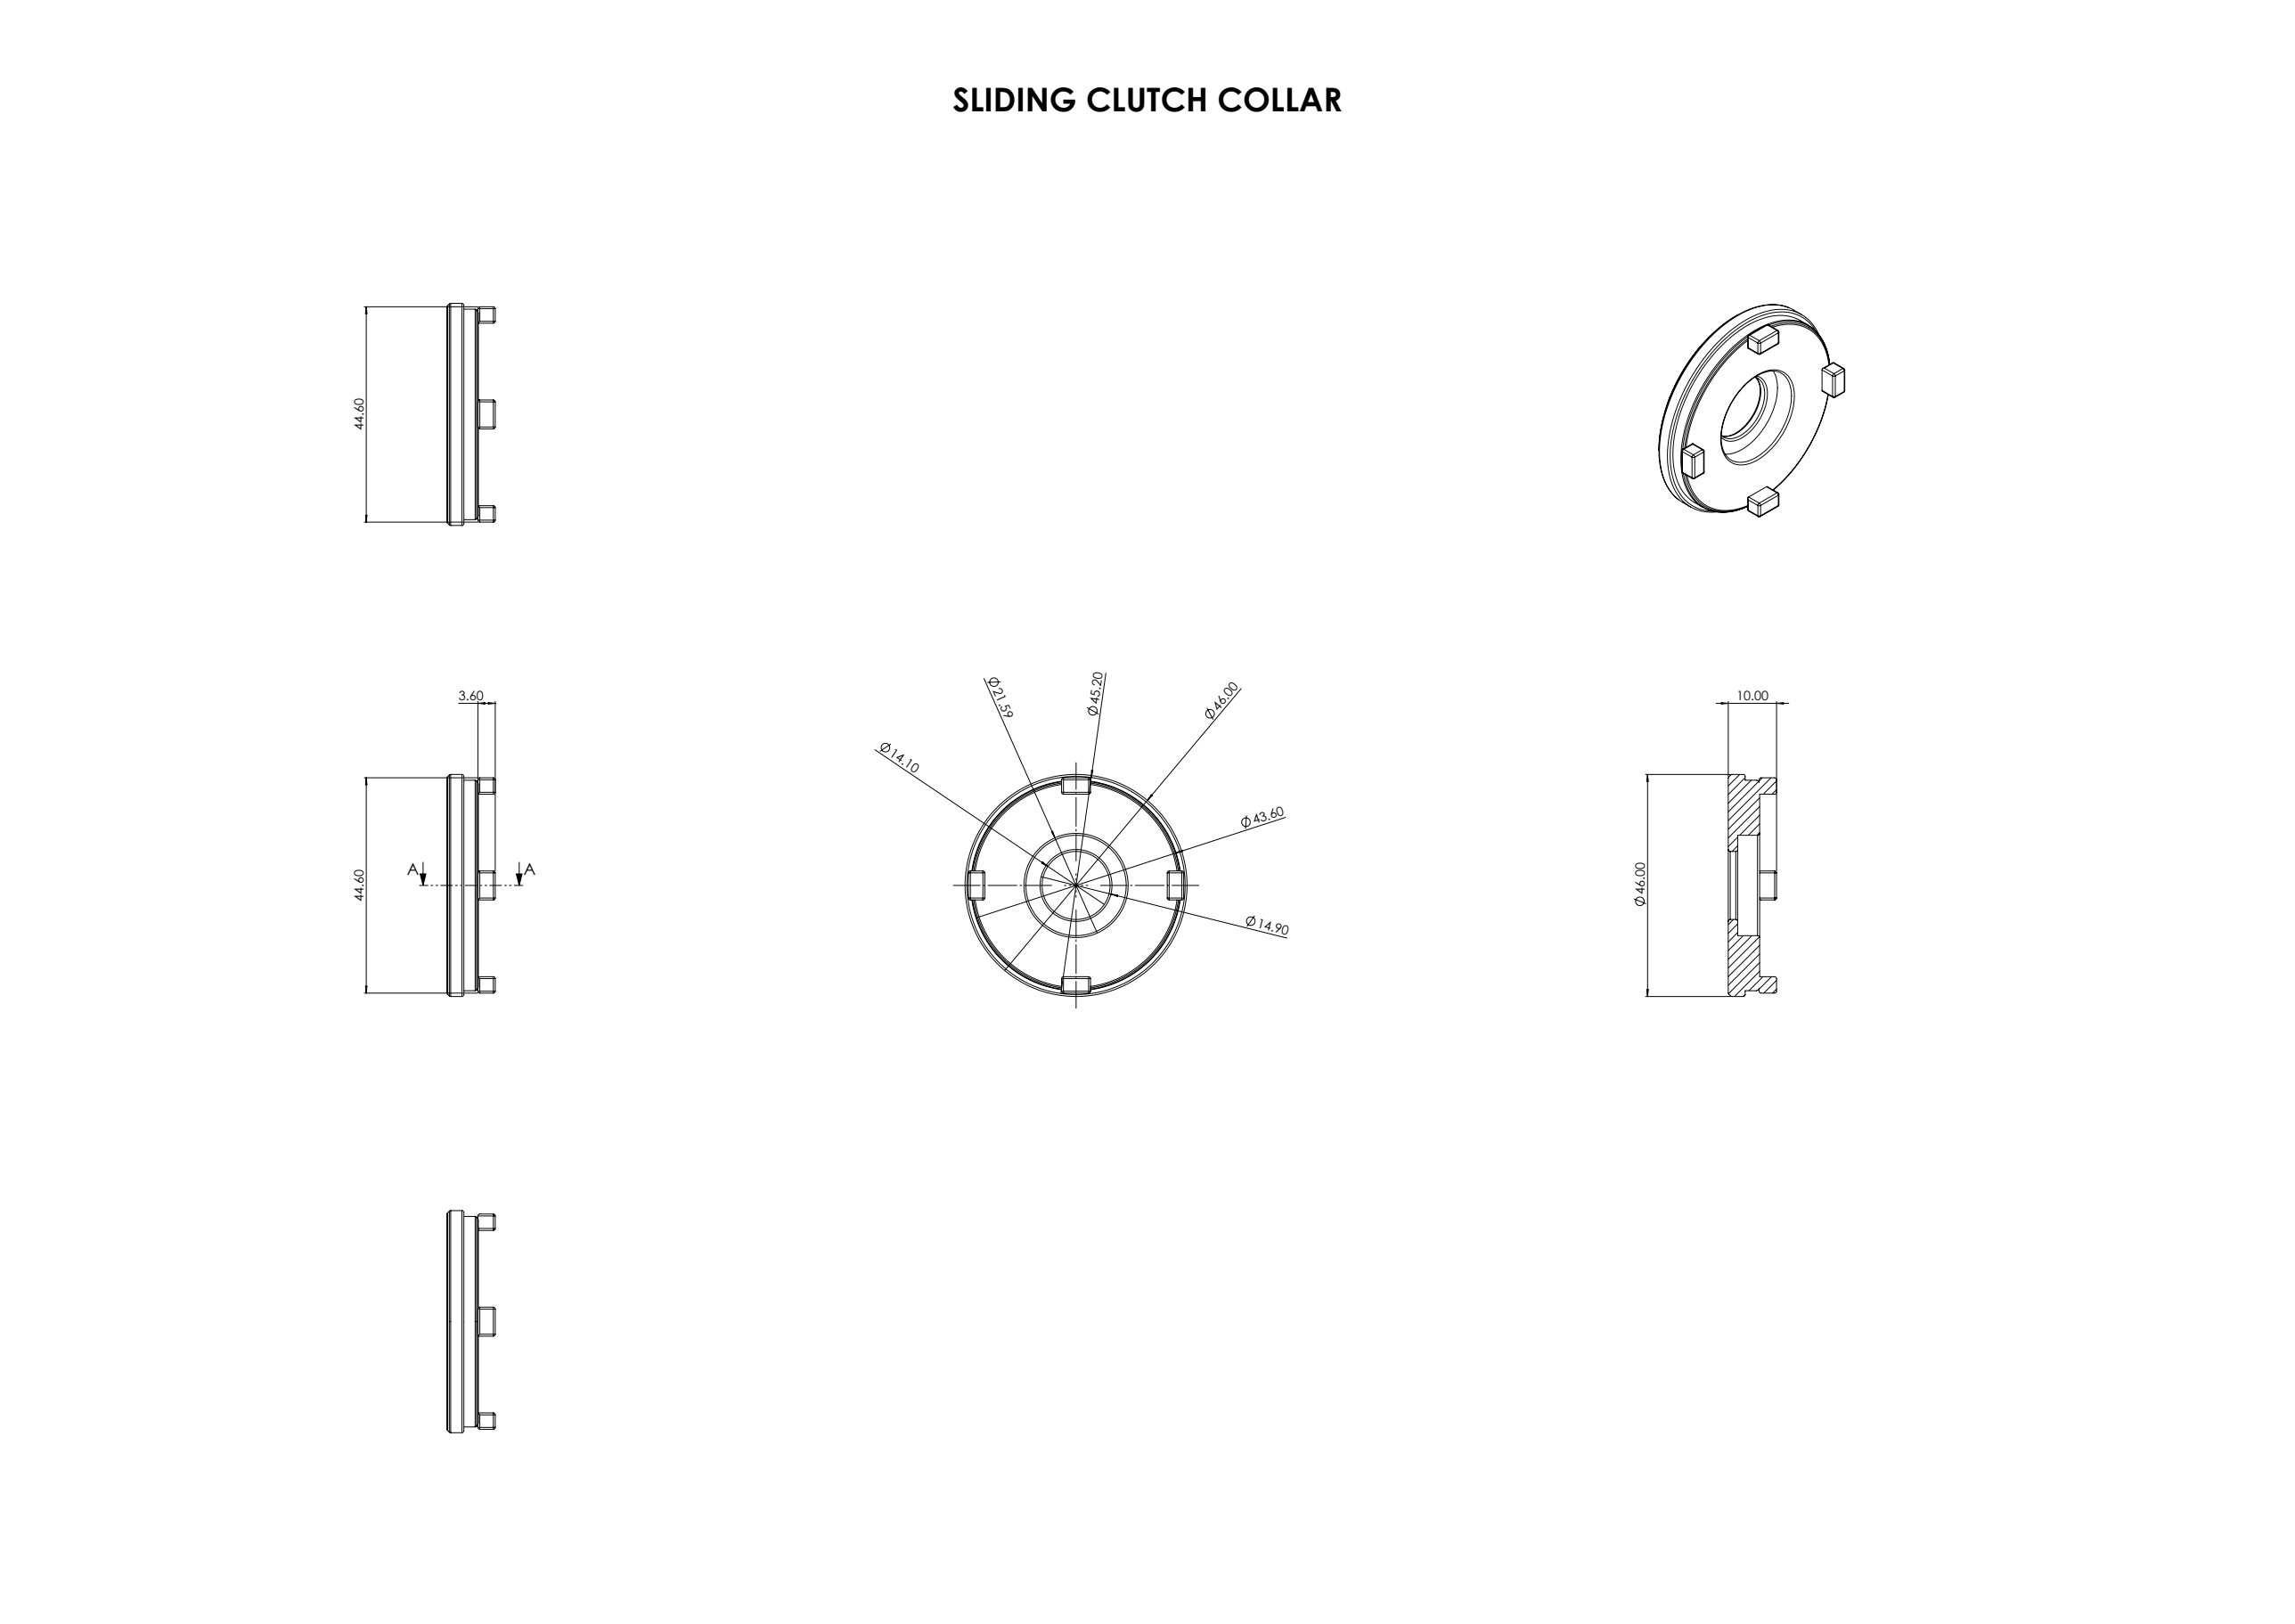
ISO-10303-21;
HEADER;
/* Generated by software containing ST-Developer
 * from STEP Tools, Inc. (www.steptools.com) 
 */

FILE_DESCRIPTION(
/* description */ (''),
/* implementation_level */ '2;1');

FILE_NAME(
/* name */ '08_Sliding_Clutch_Collar.step',
/* time_stamp */ '2026-10-11T13:00:10-07:00',
/* author */ (''),
/* organization */ (''),
/* preprocessor_version */ 'ST-DEVELOPER v20.2',
/* originating_system */ 'Autodesk Translation Framework v15.15.0.0',
/* authorisation */ '');

FILE_SCHEMA (('AUTOMOTIVE_DESIGN { 1 0 10303 214 3 1 1 }'));
ENDSEC;

DATA;
#10=MECHANICAL_DESIGN_GEOMETRIC_PRESENTATION_REPRESENTATION('',(#365),#65563);
#160=TOROIDAL_SURFACE('',#21892,21.1343145750508,0.4);
#161=TOROIDAL_SURFACE('',#21909,22.6,0.4);
#162=TOROIDAL_SURFACE('',#21951,22.6,0.4);
#163=TOROIDAL_SURFACE('',#21958,21.4,0.4);
#164=TOROIDAL_SURFACE('',#21963,10.7968626966597,0.4);
#165=TOROIDAL_SURFACE('',#21966,22.2343145750508,0.4);
#166=TOROIDAL_SURFACE('',#21990,7.45,0.4);
#167=TOROIDAL_SURFACE('',#21997,7.45,0.4);
#233=ELLIPSE('',#21780,0.565685424949238,0.4);
#234=ELLIPSE('',#21783,0.565685424949238,0.4);
#235=ELLIPSE('',#21819,0.565685424949238,0.4);
#236=ELLIPSE('',#21828,0.565685424949238,0.4);
#237=ELLIPSE('',#21872,0.565685424949238,0.4);
#238=ELLIPSE('',#21877,0.565685424949238,0.4);
#239=ELLIPSE('',#21929,0.565685424949238,0.4);
#240=ELLIPSE('',#21973,0.565685424949238,0.4);
#292=SPHERICAL_SURFACE('',#21784,0.4);
#293=SPHERICAL_SURFACE('',#21791,0.4);
#294=SPHERICAL_SURFACE('',#21794,0.4);
#295=SPHERICAL_SURFACE('',#21799,0.4);
#296=SPHERICAL_SURFACE('',#21809,0.4);
#297=SPHERICAL_SURFACE('',#21823,0.4);
#298=SPHERICAL_SURFACE('',#21831,0.4);
#299=SPHERICAL_SURFACE('',#21833,0.4);
#300=SPHERICAL_SURFACE('',#21840,0.4);
#301=SPHERICAL_SURFACE('',#21846,0.4);
#302=SPHERICAL_SURFACE('',#21859,0.4);
#303=SPHERICAL_SURFACE('',#21862,0.4);
#304=SPHERICAL_SURFACE('',#21879,0.4);
#305=SPHERICAL_SURFACE('',#21881,0.4);
#306=SPHERICAL_SURFACE('',#21919,0.4);
#307=SPHERICAL_SURFACE('',#21925,0.4);
#308=SPHERICAL_SURFACE('',#21937,0.4);
#309=SPHERICAL_SURFACE('',#21940,0.4);
#310=SPHERICAL_SURFACE('',#21942,0.4);
#311=SPHERICAL_SURFACE('',#21974,0.4);
#312=SPHERICAL_SURFACE('',#21982,0.4);
#313=SPHERICAL_SURFACE('',#21985,0.4);
#343=SHAPE_REPRESENTATION_RELATIONSHIP('SRR','None',#65621,#354);
#354=ADVANCED_BREP_SHAPE_REPRESENTATION('',(#376),#65559);
#365=STYLED_ITEM('',(#65802),#376);
#376=MANIFOLD_SOLID_BREP('Body1',#20015);
#493=CONICAL_SURFACE('',#21906,21.55,0.785398163397451);
#494=CONICAL_SURFACE('',#21955,22.7,0.785398163397452);
#984=PLANE('',#21804);
#985=PLANE('',#21805);
#986=PLANE('',#21814);
#987=PLANE('',#21815);
#988=PLANE('',#21838);
#989=PLANE('',#21852);
#990=PLANE('',#21853);
#991=PLANE('',#21869);
#992=PLANE('',#21885);
#993=PLANE('',#21886);
#994=PLANE('',#21888);
#995=PLANE('',#21902);
#996=PLANE('',#21917);
#997=PLANE('',#21926);
#998=PLANE('',#21927);
#999=PLANE('',#21944);
#1000=PLANE('',#21947);
#1001=PLANE('',#21950);
#1002=PLANE('',#21969);
#1003=PLANE('',#21978);
#1004=PLANE('',#21981);
#1005=PLANE('',#22000);
#1006=PLANE('',#22003);
#1007=PLANE('',#22004);
#1008=PLANE('',#22005);
#1009=PLANE('',#22006);
#1010=PLANE('',#22007);
#1011=PLANE('',#22008);
#1120=FACE_BOUND('',#3296,.T.);
#1121=FACE_BOUND('',#3301,.T.);
#1122=FACE_BOUND('',#3326,.T.);
#1123=FACE_BOUND('',#3342,.T.);
#2016=FACE_OUTER_BOUND('',#3240,.T.);
#2017=FACE_OUTER_BOUND('',#3241,.T.);
#2018=FACE_OUTER_BOUND('',#3242,.T.);
#2019=FACE_OUTER_BOUND('',#3243,.T.);
#2020=FACE_OUTER_BOUND('',#3244,.T.);
#2021=FACE_OUTER_BOUND('',#3245,.T.);
#2022=FACE_OUTER_BOUND('',#3246,.T.);
#2023=FACE_OUTER_BOUND('',#3247,.T.);
#2024=FACE_OUTER_BOUND('',#3248,.T.);
#2025=FACE_OUTER_BOUND('',#3249,.T.);
#2026=FACE_OUTER_BOUND('',#3250,.T.);
#2027=FACE_OUTER_BOUND('',#3251,.T.);
#2028=FACE_OUTER_BOUND('',#3252,.T.);
#2029=FACE_OUTER_BOUND('',#3253,.T.);
#2030=FACE_OUTER_BOUND('',#3254,.T.);
#2031=FACE_OUTER_BOUND('',#3255,.T.);
#2032=FACE_OUTER_BOUND('',#3256,.T.);
#2033=FACE_OUTER_BOUND('',#3257,.T.);
#2034=FACE_OUTER_BOUND('',#3258,.T.);
#2035=FACE_OUTER_BOUND('',#3259,.T.);
#2036=FACE_OUTER_BOUND('',#3260,.T.);
#2037=FACE_OUTER_BOUND('',#3261,.T.);
#2038=FACE_OUTER_BOUND('',#3262,.T.);
#2039=FACE_OUTER_BOUND('',#3263,.T.);
#2040=FACE_OUTER_BOUND('',#3264,.T.);
#2041=FACE_OUTER_BOUND('',#3265,.T.);
#2042=FACE_OUTER_BOUND('',#3266,.T.);
#2043=FACE_OUTER_BOUND('',#3267,.T.);
#2044=FACE_OUTER_BOUND('',#3268,.T.);
#2045=FACE_OUTER_BOUND('',#3269,.T.);
#2046=FACE_OUTER_BOUND('',#3270,.T.);
#2047=FACE_OUTER_BOUND('',#3271,.T.);
#2048=FACE_OUTER_BOUND('',#3272,.T.);
#2049=FACE_OUTER_BOUND('',#3273,.T.);
#2050=FACE_OUTER_BOUND('',#3274,.T.);
#2051=FACE_OUTER_BOUND('',#3275,.T.);
#2052=FACE_OUTER_BOUND('',#3276,.T.);
#2053=FACE_OUTER_BOUND('',#3277,.T.);
#2054=FACE_OUTER_BOUND('',#3278,.T.);
#2055=FACE_OUTER_BOUND('',#3279,.T.);
#2056=FACE_OUTER_BOUND('',#3280,.T.);
#2057=FACE_OUTER_BOUND('',#3281,.T.);
#2058=FACE_OUTER_BOUND('',#3282,.T.);
#2059=FACE_OUTER_BOUND('',#3283,.T.);
#2060=FACE_OUTER_BOUND('',#3284,.T.);
#2061=FACE_OUTER_BOUND('',#3285,.T.);
#2062=FACE_OUTER_BOUND('',#3286,.T.);
#2063=FACE_OUTER_BOUND('',#3287,.T.);
#2064=FACE_OUTER_BOUND('',#3288,.T.);
#2065=FACE_OUTER_BOUND('',#3289,.T.);
#2066=FACE_OUTER_BOUND('',#3290,.T.);
#2067=FACE_OUTER_BOUND('',#3291,.T.);
#2068=FACE_OUTER_BOUND('',#3292,.T.);
#2069=FACE_OUTER_BOUND('',#3293,.T.);
#2070=FACE_OUTER_BOUND('',#3294,.T.);
#2071=FACE_OUTER_BOUND('',#3295,.T.);
#2072=FACE_OUTER_BOUND('',#3297,.T.);
#2073=FACE_OUTER_BOUND('',#3298,.T.);
#2074=FACE_OUTER_BOUND('',#3299,.T.);
#2075=FACE_OUTER_BOUND('',#3300,.T.);
#2076=FACE_OUTER_BOUND('',#3302,.T.);
#2077=FACE_OUTER_BOUND('',#3303,.T.);
#2078=FACE_OUTER_BOUND('',#3304,.T.);
#2079=FACE_OUTER_BOUND('',#3305,.T.);
#2080=FACE_OUTER_BOUND('',#3306,.T.);
#2081=FACE_OUTER_BOUND('',#3307,.T.);
#2082=FACE_OUTER_BOUND('',#3308,.T.);
#2083=FACE_OUTER_BOUND('',#3309,.T.);
#2084=FACE_OUTER_BOUND('',#3310,.T.);
#2085=FACE_OUTER_BOUND('',#3311,.T.);
#2086=FACE_OUTER_BOUND('',#3312,.T.);
#2087=FACE_OUTER_BOUND('',#3313,.T.);
#2088=FACE_OUTER_BOUND('',#3314,.T.);
#2089=FACE_OUTER_BOUND('',#3315,.T.);
#2090=FACE_OUTER_BOUND('',#3316,.T.);
#2091=FACE_OUTER_BOUND('',#3317,.T.);
#2092=FACE_OUTER_BOUND('',#3318,.T.);
#2093=FACE_OUTER_BOUND('',#3319,.T.);
#2094=FACE_OUTER_BOUND('',#3320,.T.);
#2095=FACE_OUTER_BOUND('',#3321,.T.);
#2096=FACE_OUTER_BOUND('',#3322,.T.);
#2097=FACE_OUTER_BOUND('',#3323,.T.);
#2098=FACE_OUTER_BOUND('',#3324,.T.);
#2099=FACE_OUTER_BOUND('',#3325,.T.);
#2100=FACE_OUTER_BOUND('',#3327,.T.);
#2101=FACE_OUTER_BOUND('',#3328,.T.);
#2102=FACE_OUTER_BOUND('',#3329,.T.);
#2103=FACE_OUTER_BOUND('',#3330,.T.);
#2104=FACE_OUTER_BOUND('',#3331,.T.);
#2105=FACE_OUTER_BOUND('',#3332,.T.);
#2106=FACE_OUTER_BOUND('',#3333,.T.);
#2107=FACE_OUTER_BOUND('',#3334,.T.);
#2108=FACE_OUTER_BOUND('',#3335,.T.);
#2109=FACE_OUTER_BOUND('',#3336,.T.);
#2110=FACE_OUTER_BOUND('',#3337,.T.);
#2111=FACE_OUTER_BOUND('',#3338,.T.);
#2112=FACE_OUTER_BOUND('',#3339,.T.);
#2113=FACE_OUTER_BOUND('',#3340,.T.);
#2114=FACE_OUTER_BOUND('',#3341,.T.);
#2115=FACE_OUTER_BOUND('',#3343,.T.);
#2116=FACE_OUTER_BOUND('',#3344,.T.);
#2117=FACE_OUTER_BOUND('',#3345,.T.);
#2118=FACE_OUTER_BOUND('',#3346,.T.);
#2119=FACE_OUTER_BOUND('',#3347,.T.);
#2120=FACE_OUTER_BOUND('',#3348,.T.);
#2121=FACE_OUTER_BOUND('',#3349,.T.);
#3240=EDGE_LOOP('',(#16864,#16865,#16866,#16867,#16868,#16869));
#3241=EDGE_LOOP('',(#16870,#16871,#16872,#16873));
#3242=EDGE_LOOP('',(#16874,#16875,#16876));
#3243=EDGE_LOOP('',(#16877,#16878,#16879,#16880));
#3244=EDGE_LOOP('',(#16881,#16882,#16883,#16884));
#3245=EDGE_LOOP('',(#16885,#16886,#16887));
#3246=EDGE_LOOP('',(#16888,#16889,#16890));
#3247=EDGE_LOOP('',(#16891,#16892,#16893,#16894));
#3248=EDGE_LOOP('',(#16895,#16896,#16897));
#3249=EDGE_LOOP('',(#16898,#16899,#16900,#16901,#16902));
#3250=EDGE_LOOP('',(#16903,#16904,#16905,#16906));
#3251=EDGE_LOOP('',(#16907,#16908,#16909,#16910));
#3252=EDGE_LOOP('',(#16911,#16912,#16913,#16914));
#3253=EDGE_LOOP('',(#16915,#16916,#16917,#16918));
#3254=EDGE_LOOP('',(#16919,#16920,#16921));
#3255=EDGE_LOOP('',(#16922,#16923,#16924,#16925));
#3256=EDGE_LOOP('',(#16926,#16927,#16928,#16929));
#3257=EDGE_LOOP('',(#16930,#16931,#16932,#16933));
#3258=EDGE_LOOP('',(#16934,#16935,#16936,#16937));
#3259=EDGE_LOOP('',(#16938,#16939,#16940,#16941,#16942,#16943));
#3260=EDGE_LOOP('',(#16944,#16945,#16946,#16947));
#3261=EDGE_LOOP('',(#16948,#16949,#16950));
#3262=EDGE_LOOP('',(#16951,#16952,#16953,#16954));
#3263=EDGE_LOOP('',(#16955,#16956,#16957,#16958));
#3264=EDGE_LOOP('',(#16959,#16960,#16961));
#3265=EDGE_LOOP('',(#16962,#16963,#16964));
#3266=EDGE_LOOP('',(#16965,#16966,#16967,#16968,#16969));
#3267=EDGE_LOOP('',(#16970,#16971,#16972,#16973));
#3268=EDGE_LOOP('',(#16974,#16975,#16976,#16977));
#3269=EDGE_LOOP('',(#16978,#16979,#16980));
#3270=EDGE_LOOP('',(#16981,#16982,#16983,#16984));
#3271=EDGE_LOOP('',(#16985,#16986,#16987));
#3272=EDGE_LOOP('',(#16988,#16989,#16990,#16991));
#3273=EDGE_LOOP('',(#16992,#16993,#16994,#16995));
#3274=EDGE_LOOP('',(#16996,#16997,#16998,#16999));
#3275=EDGE_LOOP('',(#17000,#17001,#17002,#17003));
#3276=EDGE_LOOP('',(#17004,#17005,#17006,#17007,#17008));
#3277=EDGE_LOOP('',(#17009,#17010,#17011,#17012));
#3278=EDGE_LOOP('',(#17013,#17014,#17015));
#3279=EDGE_LOOP('',(#17016,#17017,#17018));
#3280=EDGE_LOOP('',(#17019,#17020,#17021,#17022));
#3281=EDGE_LOOP('',(#17023,#17024,#17025,#17026));
#3282=EDGE_LOOP('',(#17027,#17028,#17029,#17030));
#3283=EDGE_LOOP('',(#17031,#17032,#17033,#17034,#17035,#17036));
#3284=EDGE_LOOP('',(#17037,#17038,#17039,#17040));
#3285=EDGE_LOOP('',(#17041,#17042,#17043,#17044,#17045,#17046));
#3286=EDGE_LOOP('',(#17047,#17048,#17049));
#3287=EDGE_LOOP('',(#17050,#17051,#17052));
#3288=EDGE_LOOP('',(#17053,#17054,#17055,#17056,#17057));
#3289=EDGE_LOOP('',(#17058,#17059,#17060,#17061));
#3290=EDGE_LOOP('',(#17062,#17063,#17064,#17065));
#3291=EDGE_LOOP('',(#17066,#17067,#17068,#17069));
#3292=EDGE_LOOP('',(#17070,#17071,#17072,#17073));
#3293=EDGE_LOOP('',(#17074,#17075,#17076,#17077,#17078));
#3294=EDGE_LOOP('',(#17079,#17080,#17081,#17082,#17083,#17084,#17085,#17086,
#17087,#17088,#17089,#17090,#17091,#17092,#17093,#17094,#17095,#17096,#17097,
#17098,#17099));
#3295=EDGE_LOOP('',(#17100,#17101,#17102,#17103,#17104,#17105,#17106,#17107,
#17108,#17109,#17110,#17111,#17112,#17113,#17114,#17115,#17116,#17117,#17118,
#17119,#17120,#17121,#17122,#17123));
#3296=EDGE_LOOP('',(#17124));
#3297=EDGE_LOOP('',(#17125,#17126,#17127,#17128,#17129,#17130));
#3298=EDGE_LOOP('',(#17131,#17132,#17133,#17134,#17135));
#3299=EDGE_LOOP('',(#17136,#17137,#17138,#17139,#17140,#17141));
#3300=EDGE_LOOP('',(#17142));
#3301=EDGE_LOOP('',(#17143));
#3302=EDGE_LOOP('',(#17144,#17145,#17146));
#3303=EDGE_LOOP('',(#17147,#17148,#17149,#17150));
#3304=EDGE_LOOP('',(#17151,#17152,#17153,#17154));
#3305=EDGE_LOOP('',(#17155,#17156,#17157));
#3306=EDGE_LOOP('',(#17158,#17159,#17160,#17161));
#3307=EDGE_LOOP('',(#17162,#17163,#17164,#17165));
#3308=EDGE_LOOP('',(#17166,#17167,#17168,#17169,#17170,#17171));
#3309=EDGE_LOOP('',(#17172,#17173,#17174,#17175));
#3310=EDGE_LOOP('',(#17176,#17177,#17178,#17179));
#3311=EDGE_LOOP('',(#17180,#17181,#17182));
#3312=EDGE_LOOP('',(#17183,#17184,#17185));
#3313=EDGE_LOOP('',(#17186,#17187,#17188));
#3314=EDGE_LOOP('',(#17189,#17190,#17191,#17192));
#3315=EDGE_LOOP('',(#17193,#17194,#17195,#17196));
#3316=EDGE_LOOP('',(#17197,#17198,#17199,#17200));
#3317=EDGE_LOOP('',(#17201,#17202,#17203,#17204));
#3318=EDGE_LOOP('',(#17205,#17206,#17207,#17208));
#3319=EDGE_LOOP('',(#17209,#17210,#17211,#17212,#17213,#17214));
#3320=EDGE_LOOP('',(#17215,#17216,#17217,#17218,#17219,#17220));
#3321=EDGE_LOOP('',(#17221,#17222,#17223,#17224,#17225,#17226));
#3322=EDGE_LOOP('',(#17227,#17228,#17229,#17230,#17231));
#3323=EDGE_LOOP('',(#17232,#17233,#17234,#17235));
#3324=EDGE_LOOP('',(#17236,#17237,#17238,#17239,#17240));
#3325=EDGE_LOOP('',(#17241));
#3326=EDGE_LOOP('',(#17242));
#3327=EDGE_LOOP('',(#17243,#17244,#17245,#17246,#17247,#17248));
#3328=EDGE_LOOP('',(#17249,#17250,#17251));
#3329=EDGE_LOOP('',(#17252,#17253,#17254,#17255,#17256));
#3330=EDGE_LOOP('',(#17257,#17258,#17259,#17260));
#3331=EDGE_LOOP('',(#17261,#17262,#17263,#17264));
#3332=EDGE_LOOP('',(#17265,#17266,#17267,#17268));
#3333=EDGE_LOOP('',(#17269,#17270,#17271));
#3334=EDGE_LOOP('',(#17272,#17273,#17274,#17275,#17276));
#3335=EDGE_LOOP('',(#17277,#17278,#17279));
#3336=EDGE_LOOP('',(#17280,#17281,#17282,#17283));
#3337=EDGE_LOOP('',(#17284,#17285,#17286,#17287));
#3338=EDGE_LOOP('',(#17288,#17289,#17290,#17291,#17292));
#3339=EDGE_LOOP('',(#17293,#17294,#17295,#17296,#17297,#17298));
#3340=EDGE_LOOP('',(#17299,#17300,#17301,#17302,#17303));
#3341=EDGE_LOOP('',(#17304));
#3342=EDGE_LOOP('',(#17305));
#3343=EDGE_LOOP('',(#17306,#17307,#17308,#17309));
#3344=EDGE_LOOP('',(#17310,#17311,#17312,#17313));
#3345=EDGE_LOOP('',(#17314,#17315,#17316,#17317));
#3346=EDGE_LOOP('',(#17318,#17319,#17320,#17321,#17322,#17323));
#3347=EDGE_LOOP('',(#17324,#17325,#17326,#17327));
#3348=EDGE_LOOP('',(#17328,#17329,#17330,#17331));
#3349=EDGE_LOOP('',(#17332,#17333,#17334,#17335,#17336,#17337));
#4364=CIRCLE('',#21779,0.4);
#4365=CIRCLE('',#21782,0.4);
#4366=CIRCLE('',#21785,0.4);
#4367=CIRCLE('',#21786,0.4);
#4368=CIRCLE('',#21787,0.4);
#4369=CIRCLE('',#21790,0.4);
#4370=CIRCLE('',#21792,0.399999999999999);
#4371=CIRCLE('',#21793,0.399999999999999);
#4372=CIRCLE('',#21795,0.4);
#4373=CIRCLE('',#21796,0.4);
#4374=CIRCLE('',#21797,0.400000000000001);
#4375=CIRCLE('',#21800,0.400000000000001);
#4376=CIRCLE('',#21802,0.4);
#4377=CIRCLE('',#21803,0.4);
#4378=CIRCLE('',#21808,0.4);
#4379=CIRCLE('',#21810,0.4);
#4380=CIRCLE('',#21811,0.4);
#4381=CIRCLE('',#21816,21.3988897061572);
#4382=CIRCLE('',#21818,0.4);
#4383=CIRCLE('',#21821,0.4);
#4384=CIRCLE('',#21822,0.4);
#4385=CIRCLE('',#21824,0.4);
#4386=CIRCLE('',#21825,0.400000000000001);
#4387=CIRCLE('',#21827,0.4);
#4388=CIRCLE('',#21830,0.4);
#4389=CIRCLE('',#21832,0.4);
#4390=CIRCLE('',#21834,0.400000000000001);
#4391=CIRCLE('',#21836,0.4);
#4392=CIRCLE('',#21837,0.4);
#4393=CIRCLE('',#21841,0.4);
#4394=CIRCLE('',#21842,0.4);
#4395=CIRCLE('',#21843,0.4);
#4396=CIRCLE('',#21845,0.4);
#4397=CIRCLE('',#21847,0.4);
#4398=CIRCLE('',#21848,0.4);
#4399=CIRCLE('',#21854,21.3988897061572);
#4400=CIRCLE('',#21855,21.3988897061572);
#4401=CIRCLE('',#21857,0.4);
#4402=CIRCLE('',#21858,0.4);
#4403=CIRCLE('',#21860,0.400000000000001);
#4404=CIRCLE('',#21861,0.4);
#4405=CIRCLE('',#21863,0.4);
#4406=CIRCLE('',#21864,0.400000000000001);
#4407=CIRCLE('',#21866,0.400000000000001);
#4408=CIRCLE('',#21868,0.4);
#4409=CIRCLE('',#21871,0.4);
#4410=CIRCLE('',#21874,0.4);
#4411=CIRCLE('',#21875,0.4);
#4412=CIRCLE('',#21878,0.4);
#4413=CIRCLE('',#21880,0.400000000000001);
#4414=CIRCLE('',#21883,0.399999999999999);
#4415=CIRCLE('',#21884,0.4);
#4416=CIRCLE('',#21890,0.4);
#4417=CIRCLE('',#21891,0.4);
#4418=CIRCLE('',#21893,0.4);
#4419=CIRCLE('',#21894,21.4171572875254);
#4420=CIRCLE('',#21895,21.4171572875254);
#4421=CIRCLE('',#21896,21.1343145750508);
#4422=CIRCLE('',#21897,21.3988897061572);
#4423=CIRCLE('',#21898,21.1343145750508);
#4424=CIRCLE('',#21899,21.3988897061572);
#4425=CIRCLE('',#21900,21.1343145750508);
#4426=CIRCLE('',#21901,21.1343145750508);
#4427=CIRCLE('',#21903,0.4);
#4428=CIRCLE('',#21904,0.4);
#4429=CIRCLE('',#21905,10.7968626966597);
#4430=CIRCLE('',#21907,21.6828427124746);
#4431=CIRCLE('',#21908,21.6828427124746);
#4432=CIRCLE('',#21910,22.6);
#4433=CIRCLE('',#21911,0.4);
#4434=CIRCLE('',#21912,23.);
#4435=CIRCLE('',#21913,23.);
#4436=CIRCLE('',#21915,23.);
#4437=CIRCLE('',#21916,23.);
#4438=CIRCLE('',#21918,21.8);
#4439=CIRCLE('',#21920,0.4);
#4440=CIRCLE('',#21921,0.4);
#4441=CIRCLE('',#21923,0.4);
#4442=CIRCLE('',#21930,0.4);
#4443=CIRCLE('',#21932,0.4);
#4444=CIRCLE('',#21933,0.4);
#4445=CIRCLE('',#21935,0.4);
#4446=CIRCLE('',#21936,0.4);
#4447=CIRCLE('',#21938,0.399999999999999);
#4448=CIRCLE('',#21939,0.399999999999999);
#4449=CIRCLE('',#21941,0.400000000000001);
#4450=CIRCLE('',#21943,0.400000000000001);
#4451=CIRCLE('',#21946,0.4);
#4452=CIRCLE('',#21949,0.4);
#4453=CIRCLE('',#21952,0.4);
#4454=CIRCLE('',#21953,22.8828427124746);
#4455=CIRCLE('',#21954,22.8828427124746);
#4456=CIRCLE('',#21956,22.5171572875254);
#4457=CIRCLE('',#21957,22.5171572875254);
#4458=CIRCLE('',#21959,0.4);
#4459=CIRCLE('',#21960,21.8);
#4460=CIRCLE('',#21961,21.8);
#4461=CIRCLE('',#21964,10.4);
#4462=CIRCLE('',#21965,0.4);
#4463=CIRCLE('',#21967,0.4);
#4464=CIRCLE('',#21968,22.2343145750508);
#4465=CIRCLE('',#21970,7.45);
#4466=CIRCLE('',#21972,0.4);
#4467=CIRCLE('',#21975,0.400000000000001);
#4468=CIRCLE('',#21977,0.4);
#4469=CIRCLE('',#21980,0.400000000000001);
#4470=CIRCLE('',#21983,0.4);
#4471=CIRCLE('',#21986,0.4);
#4472=CIRCLE('',#21987,0.4);
#4473=CIRCLE('',#21991,0.4);
#4474=CIRCLE('',#21992,7.05);
#4475=CIRCLE('',#21993,7.05);
#4476=CIRCLE('',#21995,7.05);
#4477=CIRCLE('',#21996,7.05);
#4478=CIRCLE('',#21998,0.4);
#4479=CIRCLE('',#21999,7.45);
#4480=CIRCLE('',#22001,10.4);
#5348=B_SPLINE_CURVE_WITH_KNOTS('',3,(#62004,#62005,#62006,#62007,#62008,
#62009,#62010,#62011,#62012,#62013,#62014,#62015,#62016,#62017,#62018),
 .UNSPECIFIED.,.F.,.F.,(4,3,2,2,2,2,4),(-0.00329079135824289,0.,0.0066432817682188,
0.0172206827634487,0.0289541451570132,0.039919328261124,0.0424908650280393),
 .UNSPECIFIED.);
#5349=B_SPLINE_CURVE_WITH_KNOTS('',3,(#62105,#62106,#62107,#62108,#62109,
#62110,#62111,#62112,#62113,#62114,#62115,#62116,#62117,#62118,#62119),
 .UNSPECIFIED.,.F.,.F.,(4,3,2,2,2,2,4),(-0.00329079135824245,0.,0.00664328176821677,
0.0172206827634322,0.0289541451569808,0.0399193282610819,0.0424908650279941),
 .UNSPECIFIED.);
#5350=B_SPLINE_CURVE_WITH_KNOTS('',3,(#62240,#62241,#62242,#62243,#62244,
#62245,#62246,#62247,#62248,#62249,#62250,#62251,#62252,#62253,#62254),
 .UNSPECIFIED.,.F.,.F.,(4,3,2,2,2,2,4),(-0.00329079135824467,0.,0.00664328176822443,
0.0172206827634871,0.0289541451570832,0.0399193282612205,0.0424908650281417),
 .UNSPECIFIED.);
#5351=B_SPLINE_CURVE_WITH_KNOTS('',3,(#62280,#62281,#62282,#62283,#62284,
#62285,#62286,#62287,#62288,#62289,#62290,#62291,#62292,#62293,#62294),
 .UNSPECIFIED.,.F.,.F.,(4,2,2,2,3,2,4),(-0.042480297745229,-0.0324603624462188,
-0.0213862802599032,-0.0097989641520867,0.,0.00323812560369846,0.00328789213043021),
 .UNSPECIFIED.);
#5352=B_SPLINE_CURVE_WITH_KNOTS('',3,(#62323,#62324,#62325,#62326,#62327,
#62328),.UNSPECIFIED.,.F.,.F.,(4,2,4),(0.0321300733325589,0.0445286131406419,
0.0595369958610961),.UNSPECIFIED.);
#5353=B_SPLINE_CURVE_WITH_KNOTS('',3,(#62339,#62340,#62341,#62342,#62343,
#62344,#62345,#62346,#62347,#62348,#62349,#62350,#62351,#62352,#62353,#62354,
#62355,#62356,#62357,#62358,#62359),.UNSPECIFIED.,.F.,.F.,(4,2,2,2,3,2,
2,2,2,4),(0.173757899546907,0.173876480819041,0.174078751267789,0.174509383268949,
0.177045668856987,0.182861205270908,0.190817433861452,0.200151573933346,
0.210419579997881,0.219485681147617),.UNSPECIFIED.);
#5354=B_SPLINE_CURVE_WITH_KNOTS('',3,(#62363,#62364,#62365,#62366,#62367,
#62368,#62369,#62370,#62371,#62372,#62373,#62374,#62375,#62376,#62377,#62378,
#62379,#62380,#62381,#62382,#62383),.UNSPECIFIED.,.F.,.F.,(4,2,2,2,2,3,
2,2,2,4),(0.134450369378915,0.14123202266608,0.152737468233511,0.161147712982236,
0.166702035392685,0.176890070113637,0.179458084695312,0.179868341709683,
0.180066634123894,0.180178050765678),.UNSPECIFIED.);
#5355=B_SPLINE_CURVE_WITH_KNOTS('',3,(#62386,#62387,#62388,#62389,#62390,
#62391),.UNSPECIFIED.,.F.,.F.,(4,2,4),(0.0321300733325583,0.0445286131406419,
0.0595369958610961),.UNSPECIFIED.);
#6026=LINE('',#62020,#6918);
#6027=LINE('',#62024,#6919);
#6028=LINE('',#62027,#6920);
#6029=LINE('',#62031,#6921);
#6030=LINE('',#62034,#6922);
#6031=LINE('',#62044,#6923);
#6032=LINE('',#62045,#6924);
#6033=LINE('',#62050,#6925);
#6034=LINE('',#62051,#6926);
#6035=LINE('',#62064,#6927);
#6036=LINE('',#62065,#6928);
#6037=LINE('',#62070,#6929);
#6038=LINE('',#62074,#6930);
#6039=LINE('',#62077,#6931);
#6040=LINE('',#62078,#6932);
#6041=LINE('',#62080,#6933);
#6042=LINE('',#62084,#6934);
#6043=LINE('',#62087,#6935);
#6044=LINE('',#62093,#6936);
#6045=LINE('',#62095,#6937);
#6046=LINE('',#62096,#6938);
#6047=LINE('',#62101,#6939);
#6048=LINE('',#62121,#6940);
#6049=LINE('',#62125,#6941);
#6050=LINE('',#62128,#6942);
#6051=LINE('',#62134,#6943);
#6052=LINE('',#62137,#6944);
#6053=LINE('',#62145,#6945);
#6054=LINE('',#62148,#6946);
#6055=LINE('',#62152,#6947);
#6056=LINE('',#62154,#6948);
#6057=LINE('',#62161,#6949);
#6058=LINE('',#62165,#6950);
#6059=LINE('',#62168,#6951);
#6060=LINE('',#62169,#6952);
#6061=LINE('',#62171,#6953);
#6062=LINE('',#62183,#6954);
#6063=LINE('',#62184,#6955);
#6064=LINE('',#62190,#6956);
#6065=LINE('',#62192,#6957);
#6066=LINE('',#62193,#6958);
#6067=LINE('',#62195,#6959);
#6068=LINE('',#62196,#6960);
#6069=LINE('',#62203,#6961);
#6070=LINE('',#62209,#6962);
#6071=LINE('',#62212,#6963);
#6072=LINE('',#62223,#6964);
#6073=LINE('',#62226,#6965);
#6074=LINE('',#62229,#6966);
#6075=LINE('',#62232,#6967);
#6076=LINE('',#62235,#6968);
#6077=LINE('',#62236,#6969);
#6078=LINE('',#62256,#6970);
#6079=LINE('',#62259,#6971);
#6080=LINE('',#62262,#6972);
#6081=LINE('',#62266,#6973);
#6082=LINE('',#62269,#6974);
#6083=LINE('',#62275,#6975);
#6084=LINE('',#62278,#6976);
#6085=LINE('',#62295,#6977);
#6086=LINE('',#62300,#6978);
#6087=LINE('',#62304,#6979);
#6088=LINE('',#62308,#6980);
#6089=LINE('',#62310,#6981);
#6090=LINE('',#62313,#6982);
#6091=LINE('',#62314,#6983);
#6092=LINE('',#62319,#6984);
#6093=LINE('',#62395,#6985);
#6094=LINE('',#62399,#6986);
#6095=LINE('',#62402,#6987);
#6096=LINE('',#62403,#6988);
#6097=LINE('',#62404,#6989);
#6098=LINE('',#62405,#6990);
#6099=LINE('',#62406,#6991);
#6100=LINE('',#62407,#6992);
#6101=LINE('',#62412,#6993);
#6102=LINE('',#62426,#6994);
#6103=LINE('',#62438,#6995);
#6104=LINE('',#62447,#6996);
#6105=LINE('',#62450,#6997);
#6106=LINE('',#62455,#6998);
#6107=LINE('',#62458,#6999);
#6108=LINE('',#62463,#7000);
#6109=LINE('',#62466,#7001);
#6110=LINE('',#62477,#7002);
#6111=LINE('',#62478,#7003);
#6112=LINE('',#62481,#7004);
#6113=LINE('',#62485,#7005);
#6114=LINE('',#62486,#7006);
#6115=LINE('',#62489,#7007);
#6116=LINE('',#62493,#7008);
#6117=LINE('',#62494,#7009);
#6118=LINE('',#62503,#7010);
#6119=LINE('',#62514,#7011);
#6120=LINE('',#62530,#7012);
#6121=LINE('',#62536,#7013);
#6122=LINE('',#62539,#7014);
#6123=LINE('',#62542,#7015);
#6124=LINE('',#62543,#7016);
#6125=LINE('',#62547,#7017);
#6126=LINE('',#62551,#7018);
#6127=LINE('',#62557,#7019);
#6128=LINE('',#62568,#7020);
#6129=LINE('',#62578,#7021);
#6918=VECTOR('',#26263,10.);
#6919=VECTOR('',#26266,10.);
#6920=VECTOR('',#26269,10.);
#6921=VECTOR('',#26272,10.);
#6922=VECTOR('',#26275,10.);
#6923=VECTOR('',#26288,10.);
#6924=VECTOR('',#26289,10.);
#6925=VECTOR('',#26294,10.);
#6926=VECTOR('',#26295,10.);
#6927=VECTOR('',#26312,10.);
#6928=VECTOR('',#26313,10.);
#6929=VECTOR('',#26320,10.);
#6930=VECTOR('',#26323,10.);
#6931=VECTOR('',#26328,10.);
#6932=VECTOR('',#26329,10.);
#6933=VECTOR('',#26332,10.);
#6934=VECTOR('',#26337,10.);
#6935=VECTOR('',#26340,10.);
#6936=VECTOR('',#26349,10.);
#6937=VECTOR('',#26352,10.);
#6938=VECTOR('',#26353,10.);
#6939=VECTOR('',#26360,10.);
#6940=VECTOR('',#26363,10.);
#6941=VECTOR('',#26366,10.);
#6942=VECTOR('',#26369,10.);
#6943=VECTOR('',#26374,10.);
#6944=VECTOR('',#26377,10.);
#6945=VECTOR('',#26386,10.);
#6946=VECTOR('',#26389,10.);
#6947=VECTOR('',#26394,10.);
#6948=VECTOR('',#26397,10.);
#6949=VECTOR('',#26408,10.);
#6950=VECTOR('',#26411,10.);
#6951=VECTOR('',#26416,10.);
#6952=VECTOR('',#26417,10.);
#6953=VECTOR('',#26420,10.);
#6954=VECTOR('',#26433,10.);
#6955=VECTOR('',#26434,10.);
#6956=VECTOR('',#26443,10.);
#6957=VECTOR('',#26446,10.);
#6958=VECTOR('',#26447,10.);
#6959=VECTOR('',#26450,10.);
#6960=VECTOR('',#26451,10.);
#6961=VECTOR('',#26460,10.);
#6962=VECTOR('',#26465,10.);
#6963=VECTOR('',#26468,10.);
#6964=VECTOR('',#26483,10.);
#6965=VECTOR('',#26486,10.);
#6966=VECTOR('',#26489,10.);
#6967=VECTOR('',#26492,10.);
#6968=VECTOR('',#26495,10.);
#6969=VECTOR('',#26496,10.);
#6970=VECTOR('',#26499,10.);
#6971=VECTOR('',#26502,10.);
#6972=VECTOR('',#26505,10.);
#6973=VECTOR('',#26510,10.);
#6974=VECTOR('',#26513,10.);
#6975=VECTOR('',#26518,10.);
#6976=VECTOR('',#26521,10.);
#6977=VECTOR('',#26522,10.);
#6978=VECTOR('',#26531,10.);
#6979=VECTOR('',#26534,10.);
#6980=VECTOR('',#26541,10.);
#6981=VECTOR('',#26544,10.);
#6982=VECTOR('',#26547,10.);
#6983=VECTOR('',#26548,10.);
#6984=VECTOR('',#26553,10.);
#6985=VECTOR('',#26578,10.);
#6986=VECTOR('',#26581,10.);
#6987=VECTOR('',#26584,10.);
#6988=VECTOR('',#26585,10.);
#6989=VECTOR('',#26586,10.);
#6990=VECTOR('',#26587,10.);
#6991=VECTOR('',#26588,10.);
#6992=VECTOR('',#26589,10.);
#6993=VECTOR('',#26594,21.55);
#6994=VECTOR('',#26611,23.);
#6995=VECTOR('',#26630,10.);
#6996=VECTOR('',#26643,10.);
#6997=VECTOR('',#26646,10.);
#6998=VECTOR('',#26651,10.);
#6999=VECTOR('',#26654,10.);
#7000=VECTOR('',#26659,10.);
#7001=VECTOR('',#26662,10.);
#7002=VECTOR('',#26679,10.);
#7003=VECTOR('',#26680,10.);
#7004=VECTOR('',#26683,10.);
#7005=VECTOR('',#26688,10.);
#7006=VECTOR('',#26689,10.);
#7007=VECTOR('',#26692,10.);
#7008=VECTOR('',#26697,10.);
#7009=VECTOR('',#26698,10.);
#7010=VECTOR('',#26709,22.7);
#7011=VECTOR('',#26724,21.8);
#7012=VECTOR('',#26745,10.);
#7013=VECTOR('',#26754,10.);
#7014=VECTOR('',#26757,10.);
#7015=VECTOR('',#26760,10.);
#7016=VECTOR('',#26761,10.);
#7017=VECTOR('',#26768,10.);
#7018=VECTOR('',#26775,10.);
#7019=VECTOR('',#26786,10.);
#7020=VECTOR('',#26799,7.05);
#7021=VECTOR('',#26814,10.4);
#8698=VERTEX_POINT('',#62002);
#8699=VERTEX_POINT('',#62003);
#8700=VERTEX_POINT('',#62019);
#8701=VERTEX_POINT('',#62021);
#8702=VERTEX_POINT('',#62023);
#8703=VERTEX_POINT('',#62025);
#8704=VERTEX_POINT('',#62029);
#8705=VERTEX_POINT('',#62030);
#8706=VERTEX_POINT('',#62033);
#8707=VERTEX_POINT('',#62037);
#8708=VERTEX_POINT('',#62038);
#8709=VERTEX_POINT('',#62040);
#8710=VERTEX_POINT('',#62047);
#8711=VERTEX_POINT('',#62048);
#8712=VERTEX_POINT('',#62053);
#8713=VERTEX_POINT('',#62057);
#8714=VERTEX_POINT('',#62058);
#8715=VERTEX_POINT('',#62060);
#8716=VERTEX_POINT('',#62069);
#8717=VERTEX_POINT('',#62071);
#8718=VERTEX_POINT('',#62073);
#8719=VERTEX_POINT('',#62083);
#8720=VERTEX_POINT('',#62085);
#8721=VERTEX_POINT('',#62089);
#8722=VERTEX_POINT('',#62099);
#8723=VERTEX_POINT('',#62103);
#8724=VERTEX_POINT('',#62104);
#8725=VERTEX_POINT('',#62120);
#8726=VERTEX_POINT('',#62122);
#8727=VERTEX_POINT('',#62124);
#8728=VERTEX_POINT('',#62126);
#8729=VERTEX_POINT('',#62130);
#8730=VERTEX_POINT('',#62131);
#8731=VERTEX_POINT('',#62133);
#8732=VERTEX_POINT('',#62135);
#8733=VERTEX_POINT('',#62139);
#8734=VERTEX_POINT('',#62143);
#8735=VERTEX_POINT('',#62144);
#8736=VERTEX_POINT('',#62147);
#8737=VERTEX_POINT('',#62151);
#8738=VERTEX_POINT('',#62160);
#8739=VERTEX_POINT('',#62162);
#8740=VERTEX_POINT('',#62164);
#8741=VERTEX_POINT('',#62173);
#8742=VERTEX_POINT('',#62174);
#8743=VERTEX_POINT('',#62176);
#8744=VERTEX_POINT('',#62180);
#8745=VERTEX_POINT('',#62181);
#8746=VERTEX_POINT('',#62186);
#8747=VERTEX_POINT('',#62199);
#8748=VERTEX_POINT('',#62201);
#8749=VERTEX_POINT('',#62205);
#8750=VERTEX_POINT('',#62206);
#8751=VERTEX_POINT('',#62208);
#8752=VERTEX_POINT('',#62210);
#8753=VERTEX_POINT('',#62214);
#8754=VERTEX_POINT('',#62218);
#8755=VERTEX_POINT('',#62222);
#8756=VERTEX_POINT('',#62224);
#8757=VERTEX_POINT('',#62228);
#8758=VERTEX_POINT('',#62230);
#8759=VERTEX_POINT('',#62234);
#8760=VERTEX_POINT('',#62238);
#8761=VERTEX_POINT('',#62239);
#8762=VERTEX_POINT('',#62255);
#8763=VERTEX_POINT('',#62258);
#8764=VERTEX_POINT('',#62260);
#8765=VERTEX_POINT('',#62265);
#8766=VERTEX_POINT('',#62267);
#8767=VERTEX_POINT('',#62271);
#8768=VERTEX_POINT('',#62272);
#8769=VERTEX_POINT('',#62274);
#8770=VERTEX_POINT('',#62277);
#8771=VERTEX_POINT('',#62279);
#8772=VERTEX_POINT('',#62301);
#8773=VERTEX_POINT('',#62303);
#8774=VERTEX_POINT('',#62312);
#8775=VERTEX_POINT('',#62316);
#8776=VERTEX_POINT('',#62318);
#8777=VERTEX_POINT('',#62322);
#8778=VERTEX_POINT('',#62329);
#8779=VERTEX_POINT('',#62331);
#8780=VERTEX_POINT('',#62336);
#8781=VERTEX_POINT('',#62338);
#8782=VERTEX_POINT('',#62360);
#8783=VERTEX_POINT('',#62362);
#8784=VERTEX_POINT('',#62384);
#8785=VERTEX_POINT('',#62394);
#8786=VERTEX_POINT('',#62396);
#8787=VERTEX_POINT('',#62398);
#8788=VERTEX_POINT('',#62400);
#8789=VERTEX_POINT('',#62408);
#8790=VERTEX_POINT('',#62411);
#8791=VERTEX_POINT('',#62413);
#8792=VERTEX_POINT('',#62417);
#8793=VERTEX_POINT('',#62419);
#8794=VERTEX_POINT('',#62421);
#8795=VERTEX_POINT('',#62425);
#8796=VERTEX_POINT('',#62427);
#8797=VERTEX_POINT('',#62431);
#8798=VERTEX_POINT('',#62444);
#8799=VERTEX_POINT('',#62446);
#8800=VERTEX_POINT('',#62448);
#8801=VERTEX_POINT('',#62452);
#8802=VERTEX_POINT('',#62454);
#8803=VERTEX_POINT('',#62456);
#8804=VERTEX_POINT('',#62460);
#8805=VERTEX_POINT('',#62462);
#8806=VERTEX_POINT('',#62464);
#8807=VERTEX_POINT('',#62468);
#8808=VERTEX_POINT('',#62476);
#8809=VERTEX_POINT('',#62480);
#8810=VERTEX_POINT('',#62484);
#8811=VERTEX_POINT('',#62488);
#8812=VERTEX_POINT('',#62492);
#8813=VERTEX_POINT('',#62496);
#8814=VERTEX_POINT('',#62498);
#8815=VERTEX_POINT('',#62502);
#8816=VERTEX_POINT('',#62504);
#8817=VERTEX_POINT('',#62508);
#8818=VERTEX_POINT('',#62510);
#8819=VERTEX_POINT('',#62516);
#8820=VERTEX_POINT('',#62520);
#8821=VERTEX_POINT('',#62524);
#8822=VERTEX_POINT('',#62527);
#8823=VERTEX_POINT('',#62529);
#8824=VERTEX_POINT('',#62535);
#8825=VERTEX_POINT('',#62537);
#8826=VERTEX_POINT('',#62541);
#8827=VERTEX_POINT('',#62559);
#8828=VERTEX_POINT('',#62561);
#8829=VERTEX_POINT('',#62565);
#8830=VERTEX_POINT('',#62566);
#8831=VERTEX_POINT('',#62571);
#8832=VERTEX_POINT('',#62575);
#11465=EDGE_CURVE('',#8698,#8699,#5348,.T.);
#11466=EDGE_CURVE('',#8698,#8700,#6026,.T.);
#11467=EDGE_CURVE('',#8700,#8701,#4364,.T.);
#11468=EDGE_CURVE('',#8701,#8702,#6027,.T.);
#11469=EDGE_CURVE('',#8702,#8703,#233,.T.);
#11470=EDGE_CURVE('',#8699,#8703,#6028,.T.);
#11471=EDGE_CURVE('',#8704,#8705,#6029,.T.);
#11472=EDGE_CURVE('',#8705,#8700,#4365,.T.);
#11473=EDGE_CURVE('',#8700,#8706,#6030,.T.);
#11474=EDGE_CURVE('',#8706,#8704,#234,.T.);
#11475=EDGE_CURVE('',#8707,#8708,#4366,.F.);
#11476=EDGE_CURVE('',#8709,#8707,#4367,.F.);
#11477=EDGE_CURVE('',#8708,#8709,#4368,.F.);
#11478=EDGE_CURVE('',#8706,#8709,#6031,.T.);
#11479=EDGE_CURVE('',#8707,#8704,#6032,.T.);
#11480=EDGE_CURVE('',#8710,#8711,#4369,.T.);
#11481=EDGE_CURVE('',#8711,#8708,#6033,.T.);
#11482=EDGE_CURVE('',#8709,#8710,#6034,.T.);
#11483=EDGE_CURVE('',#8710,#8712,#4370,.T.);
#11484=EDGE_CURVE('',#8712,#8711,#4371,.T.);
#11485=EDGE_CURVE('',#8713,#8714,#4372,.T.);
#11486=EDGE_CURVE('',#8714,#8715,#4373,.T.);
#11487=EDGE_CURVE('',#8715,#8713,#4374,.T.);
#11488=EDGE_CURVE('',#8713,#8707,#6035,.T.);
#11489=EDGE_CURVE('',#8708,#8714,#6036,.T.);
#11490=EDGE_CURVE('',#8705,#8701,#4375,.T.);
#11491=EDGE_CURVE('',#8702,#8716,#6037,.T.);
#11492=EDGE_CURVE('',#8716,#8717,#4376,.F.);
#11493=EDGE_CURVE('',#8717,#8718,#6038,.T.);
#11494=EDGE_CURVE('',#8718,#8703,#4377,.F.);
#11495=EDGE_CURVE('',#8715,#8701,#6039,.T.);
#11496=EDGE_CURVE('',#8716,#8715,#6040,.T.);
#11497=EDGE_CURVE('',#8705,#8713,#6041,.T.);
#11498=EDGE_CURVE('',#8710,#8719,#6042,.T.);
#11499=EDGE_CURVE('',#8719,#8720,#4378,.F.);
#11500=EDGE_CURVE('',#8720,#8712,#6043,.T.);
#11501=EDGE_CURVE('',#8717,#8721,#4379,.F.);
#11502=EDGE_CURVE('',#8721,#8716,#4380,.F.);
#11503=EDGE_CURVE('',#8714,#8721,#6044,.T.);
#11504=EDGE_CURVE('',#8712,#8717,#6045,.T.);
#11505=EDGE_CURVE('',#8721,#8711,#6046,.T.);
#11506=EDGE_CURVE('',#8698,#8722,#4381,.T.);
#11507=EDGE_CURVE('',#8722,#8706,#6047,.F.);
#11508=EDGE_CURVE('',#8723,#8724,#5349,.T.);
#11509=EDGE_CURVE('',#8723,#8725,#6048,.T.);
#11510=EDGE_CURVE('',#8725,#8726,#4382,.T.);
#11511=EDGE_CURVE('',#8726,#8727,#6049,.T.);
#11512=EDGE_CURVE('',#8727,#8728,#235,.T.);
#11513=EDGE_CURVE('',#8724,#8728,#6050,.T.);
#11514=EDGE_CURVE('',#8729,#8730,#4383,.T.);
#11515=EDGE_CURVE('',#8730,#8731,#6051,.T.);
#11516=EDGE_CURVE('',#8731,#8732,#4384,.T.);
#11517=EDGE_CURVE('',#8732,#8729,#6052,.T.);
#11518=EDGE_CURVE('',#8731,#8733,#4385,.T.);
#11519=EDGE_CURVE('',#8733,#8732,#4386,.T.);
#11520=EDGE_CURVE('',#8734,#8735,#6053,.T.);
#11521=EDGE_CURVE('',#8735,#8725,#4387,.T.);
#11522=EDGE_CURVE('',#8725,#8736,#6054,.T.);
#11523=EDGE_CURVE('',#8736,#8734,#236,.T.);
#11524=EDGE_CURVE('',#8736,#8737,#6055,.T.);
#11525=EDGE_CURVE('',#8737,#8729,#4388,.T.);
#11526=EDGE_CURVE('',#8729,#8734,#6056,.T.);
#11527=EDGE_CURVE('',#8737,#8730,#4389,.T.);
#11528=EDGE_CURVE('',#8735,#8726,#4390,.T.);
#11529=EDGE_CURVE('',#8727,#8738,#6057,.T.);
#11530=EDGE_CURVE('',#8738,#8739,#4391,.F.);
#11531=EDGE_CURVE('',#8739,#8740,#6058,.T.);
#11532=EDGE_CURVE('',#8740,#8728,#4392,.F.);
#11533=EDGE_CURVE('',#8733,#8726,#6059,.T.);
#11534=EDGE_CURVE('',#8738,#8733,#6060,.T.);
#11535=EDGE_CURVE('',#8735,#8732,#6061,.T.);
#11536=EDGE_CURVE('',#8741,#8742,#4393,.F.);
#11537=EDGE_CURVE('',#8743,#8741,#4394,.F.);
#11538=EDGE_CURVE('',#8742,#8743,#4395,.F.);
#11539=EDGE_CURVE('',#8744,#8745,#4396,.F.);
#11540=EDGE_CURVE('',#8745,#8743,#6062,.T.);
#11541=EDGE_CURVE('',#8741,#8744,#6063,.T.);
#11542=EDGE_CURVE('',#8739,#8746,#4397,.F.);
#11543=EDGE_CURVE('',#8746,#8738,#4398,.F.);
#11544=EDGE_CURVE('',#8731,#8746,#6064,.T.);
#11545=EDGE_CURVE('',#8746,#8742,#6065,.T.);
#11546=EDGE_CURVE('',#8743,#8739,#6066,.T.);
#11547=EDGE_CURVE('',#8737,#8741,#6067,.T.);
#11548=EDGE_CURVE('',#8742,#8730,#6068,.T.);
#11549=EDGE_CURVE('',#8723,#8747,#4399,.T.);
#11550=EDGE_CURVE('',#8747,#8748,#4400,.T.);
#11551=EDGE_CURVE('',#8748,#8736,#6069,.F.);
#11552=EDGE_CURVE('',#8749,#8750,#4401,.T.);
#11553=EDGE_CURVE('',#8750,#8751,#6070,.T.);
#11554=EDGE_CURVE('',#8751,#8752,#4402,.T.);
#11555=EDGE_CURVE('',#8752,#8749,#6071,.T.);
#11556=EDGE_CURVE('',#8751,#8753,#4403,.T.);
#11557=EDGE_CURVE('',#8753,#8752,#4404,.T.);
#11558=EDGE_CURVE('',#8749,#8754,#4405,.T.);
#11559=EDGE_CURVE('',#8754,#8750,#4406,.T.);
#11560=EDGE_CURVE('',#8754,#8755,#6072,.T.);
#11561=EDGE_CURVE('',#8756,#8755,#4407,.T.);
#11562=EDGE_CURVE('',#8756,#8750,#6073,.T.);
#11563=EDGE_CURVE('',#8749,#8757,#6074,.T.);
#11564=EDGE_CURVE('',#8757,#8758,#4408,.T.);
#11565=EDGE_CURVE('',#8758,#8754,#6075,.T.);
#11566=EDGE_CURVE('',#8759,#8752,#6076,.T.);
#11567=EDGE_CURVE('',#8757,#8759,#6077,.T.);
#11568=EDGE_CURVE('',#8760,#8761,#5350,.T.);
#11569=EDGE_CURVE('',#8760,#8762,#6078,.T.);
#11570=EDGE_CURVE('',#8762,#8755,#4409,.T.);
#11571=EDGE_CURVE('',#8755,#8763,#6079,.T.);
#11572=EDGE_CURVE('',#8763,#8764,#237,.T.);
#11573=EDGE_CURVE('',#8761,#8764,#6080,.T.);
#11574=EDGE_CURVE('',#8756,#8762,#4410,.T.);
#11575=EDGE_CURVE('',#8762,#8765,#6081,.T.);
#11576=EDGE_CURVE('',#8765,#8766,#4411,.T.);
#11577=EDGE_CURVE('',#8766,#8756,#6082,.T.);
#11578=EDGE_CURVE('',#8767,#8768,#238,.T.);
#11579=EDGE_CURVE('',#8768,#8769,#6083,.T.);
#11580=EDGE_CURVE('',#8769,#8765,#4412,.T.);
#11581=EDGE_CURVE('',#8765,#8770,#6084,.T.);
#11582=EDGE_CURVE('',#8770,#8771,#5351,.F.);
#11583=EDGE_CURVE('',#8771,#8767,#6085,.F.);
#11584=EDGE_CURVE('',#8769,#8766,#4413,.T.);
#11585=EDGE_CURVE('',#8763,#8758,#6086,.T.);
#11586=EDGE_CURVE('',#8772,#8758,#4414,.T.);
#11587=EDGE_CURVE('',#8772,#8773,#6087,.T.);
#11588=EDGE_CURVE('',#8773,#8764,#4415,.F.);
#11589=EDGE_CURVE('',#8751,#8766,#6088,.T.);
#11590=EDGE_CURVE('',#8769,#8753,#6089,.T.);
#11591=EDGE_CURVE('',#8774,#8768,#6090,.T.);
#11592=EDGE_CURVE('',#8753,#8774,#6091,.T.);
#11593=EDGE_CURVE('',#8767,#8775,#4416,.F.);
#11594=EDGE_CURVE('',#8775,#8776,#6092,.T.);
#11595=EDGE_CURVE('',#8776,#8774,#4417,.F.);
#11596=EDGE_CURVE('',#8748,#8777,#5352,.T.);
#11597=EDGE_CURVE('',#8747,#8778,#4418,.T.);
#11598=EDGE_CURVE('',#8778,#8779,#4419,.T.);
#11599=EDGE_CURVE('',#8779,#8778,#4420,.T.);
#11600=EDGE_CURVE('',#8771,#8724,#4421,.T.);
#11601=EDGE_CURVE('',#8770,#8760,#4422,.F.);
#11602=EDGE_CURVE('',#8780,#8761,#4423,.T.);
#11603=EDGE_CURVE('',#8780,#8781,#5353,.F.);
#11604=EDGE_CURVE('',#8781,#8782,#4424,.F.);
#11605=EDGE_CURVE('',#8783,#8782,#5354,.T.);
#11606=EDGE_CURVE('',#8783,#8784,#4425,.T.);
#11607=EDGE_CURVE('',#8722,#8784,#5355,.T.);
#11608=EDGE_CURVE('',#8777,#8699,#4426,.T.);
#11609=EDGE_CURVE('',#8783,#8785,#6093,.T.);
#11610=EDGE_CURVE('',#8786,#8785,#4427,.F.);
#11611=EDGE_CURVE('',#8786,#8787,#6094,.T.);
#11612=EDGE_CURVE('',#8788,#8787,#4428,.F.);
#11613=EDGE_CURVE('',#8780,#8788,#6095,.F.);
#11614=EDGE_CURVE('',#8773,#8775,#6096,.T.);
#11615=EDGE_CURVE('',#8740,#8745,#6097,.T.);
#11616=EDGE_CURVE('',#8744,#8777,#6098,.T.);
#11617=EDGE_CURVE('',#8718,#8720,#6099,.T.);
#11618=EDGE_CURVE('',#8719,#8784,#6100,.T.);
#11619=EDGE_CURVE('',#8789,#8789,#4429,.T.);
#11620=EDGE_CURVE('',#8779,#8790,#6101,.T.);
#11621=EDGE_CURVE('',#8791,#8790,#4430,.T.);
#11622=EDGE_CURVE('',#8790,#8791,#4431,.T.);
#11623=EDGE_CURVE('',#8792,#8792,#4432,.T.);
#11624=EDGE_CURVE('',#8792,#8793,#4433,.T.);
#11625=EDGE_CURVE('',#8793,#8794,#4434,.T.);
#11626=EDGE_CURVE('',#8794,#8793,#4435,.T.);
#11627=EDGE_CURVE('',#8794,#8795,#6102,.T.);
#11628=EDGE_CURVE('',#8796,#8795,#4436,.T.);
#11629=EDGE_CURVE('',#8795,#8796,#4437,.T.);
#11630=EDGE_CURVE('',#8797,#8797,#4438,.T.);
#11631=EDGE_CURVE('',#8774,#8759,#4439,.F.);
#11632=EDGE_CURVE('',#8759,#8776,#4440,.F.);
#11633=EDGE_CURVE('',#8772,#8757,#4441,.T.);
#11634=EDGE_CURVE('',#8776,#8772,#6103,.T.);
#11635=EDGE_CURVE('',#8788,#8798,#239,.T.);
#11636=EDGE_CURVE('',#8798,#8799,#6104,.T.);
#11637=EDGE_CURVE('',#8799,#8800,#4442,.T.);
#11638=EDGE_CURVE('',#8800,#8781,#6105,.T.);
#11639=EDGE_CURVE('',#8801,#8799,#4443,.T.);
#11640=EDGE_CURVE('',#8799,#8802,#6106,.T.);
#11641=EDGE_CURVE('',#8802,#8803,#4444,.T.);
#11642=EDGE_CURVE('',#8803,#8801,#6107,.T.);
#11643=EDGE_CURVE('',#8804,#8802,#4445,.T.);
#11644=EDGE_CURVE('',#8802,#8805,#6108,.T.);
#11645=EDGE_CURVE('',#8805,#8806,#4446,.T.);
#11646=EDGE_CURVE('',#8806,#8804,#6109,.T.);
#11647=EDGE_CURVE('',#8805,#8807,#4447,.T.);
#11648=EDGE_CURVE('',#8807,#8806,#4448,.T.);
#11649=EDGE_CURVE('',#8804,#8803,#4449,.T.);
#11650=EDGE_CURVE('',#8801,#8800,#4450,.T.);
#11651=EDGE_CURVE('',#8808,#8800,#6110,.T.);
#11652=EDGE_CURVE('',#8782,#8808,#6111,.T.);
#11653=EDGE_CURVE('',#8801,#8809,#6112,.T.);
#11654=EDGE_CURVE('',#8809,#8808,#4451,.T.);
#11655=EDGE_CURVE('',#8810,#8803,#6113,.T.);
#11656=EDGE_CURVE('',#8809,#8810,#6114,.T.);
#11657=EDGE_CURVE('',#8804,#8811,#6115,.T.);
#11658=EDGE_CURVE('',#8810,#8811,#4452,.T.);
#11659=EDGE_CURVE('',#8812,#8806,#6116,.T.);
#11660=EDGE_CURVE('',#8811,#8812,#6117,.T.);
#11661=EDGE_CURVE('',#8796,#8813,#4453,.T.);
#11662=EDGE_CURVE('',#8813,#8814,#4454,.T.);
#11663=EDGE_CURVE('',#8814,#8813,#4455,.T.);
#11664=EDGE_CURVE('',#8814,#8815,#6118,.T.);
#11665=EDGE_CURVE('',#8816,#8815,#4456,.T.);
#11666=EDGE_CURVE('',#8815,#8816,#4457,.T.);
#11667=EDGE_CURVE('',#8791,#8817,#4458,.T.);
#11668=EDGE_CURVE('',#8817,#8818,#4459,.T.);
#11669=EDGE_CURVE('',#8818,#8817,#4460,.T.);
#11670=EDGE_CURVE('',#8818,#8797,#6119,.T.);
#11671=EDGE_CURVE('',#8819,#8819,#4461,.T.);
#11672=EDGE_CURVE('',#8819,#8789,#4462,.T.);
#11673=EDGE_CURVE('',#8816,#8820,#4463,.T.);
#11674=EDGE_CURVE('',#8820,#8820,#4464,.T.);
#11675=EDGE_CURVE('',#8821,#8821,#4465,.T.);
#11676=EDGE_CURVE('',#8808,#8822,#4466,.T.);
#11677=EDGE_CURVE('',#8822,#8823,#6120,.T.);
#11678=EDGE_CURVE('',#8823,#8785,#240,.T.);
#11679=EDGE_CURVE('',#8809,#8822,#4467,.T.);
#11680=EDGE_CURVE('',#8823,#8824,#6121,.T.);
#11681=EDGE_CURVE('',#8824,#8825,#4468,.F.);
#11682=EDGE_CURVE('',#8825,#8786,#6122,.T.);
#11683=EDGE_CURVE('',#8826,#8822,#6123,.T.);
#11684=EDGE_CURVE('',#8824,#8826,#6124,.T.);
#11685=EDGE_CURVE('',#8826,#8810,#4469,.T.);
#11686=EDGE_CURVE('',#8805,#8798,#6125,.T.);
#11687=EDGE_CURVE('',#8811,#8826,#4470,.T.);
#11688=EDGE_CURVE('',#8787,#8807,#6126,.T.);
#11689=EDGE_CURVE('',#8825,#8812,#4471,.F.);
#11690=EDGE_CURVE('',#8812,#8824,#4472,.F.);
#11691=EDGE_CURVE('',#8807,#8825,#6127,.T.);
#11692=EDGE_CURVE('',#8821,#8827,#4473,.T.);
#11693=EDGE_CURVE('',#8827,#8828,#4474,.T.);
#11694=EDGE_CURVE('',#8828,#8827,#4475,.T.);
#11695=EDGE_CURVE('',#8829,#8830,#4476,.T.);
#11696=EDGE_CURVE('',#8829,#8828,#6128,.T.);
#11697=EDGE_CURVE('',#8830,#8829,#4477,.T.);
#11698=EDGE_CURVE('',#8830,#8831,#4478,.T.);
#11699=EDGE_CURVE('',#8831,#8831,#4479,.T.);
#11700=EDGE_CURVE('',#8832,#8832,#4480,.T.);
#11701=EDGE_CURVE('',#8832,#8819,#6129,.T.);
#16864=ORIENTED_EDGE('',*,*,#11465,.F.);
#16865=ORIENTED_EDGE('',*,*,#11466,.T.);
#16866=ORIENTED_EDGE('',*,*,#11467,.T.);
#16867=ORIENTED_EDGE('',*,*,#11468,.T.);
#16868=ORIENTED_EDGE('',*,*,#11469,.T.);
#16869=ORIENTED_EDGE('',*,*,#11470,.F.);
#16870=ORIENTED_EDGE('',*,*,#11471,.T.);
#16871=ORIENTED_EDGE('',*,*,#11472,.T.);
#16872=ORIENTED_EDGE('',*,*,#11473,.T.);
#16873=ORIENTED_EDGE('',*,*,#11474,.T.);
#16874=ORIENTED_EDGE('',*,*,#11475,.F.);
#16875=ORIENTED_EDGE('',*,*,#11476,.F.);
#16876=ORIENTED_EDGE('',*,*,#11477,.F.);
#16877=ORIENTED_EDGE('',*,*,#11478,.T.);
#16878=ORIENTED_EDGE('',*,*,#11476,.T.);
#16879=ORIENTED_EDGE('',*,*,#11479,.T.);
#16880=ORIENTED_EDGE('',*,*,#11474,.F.);
#16881=ORIENTED_EDGE('',*,*,#11480,.T.);
#16882=ORIENTED_EDGE('',*,*,#11481,.T.);
#16883=ORIENTED_EDGE('',*,*,#11477,.T.);
#16884=ORIENTED_EDGE('',*,*,#11482,.T.);
#16885=ORIENTED_EDGE('',*,*,#11480,.F.);
#16886=ORIENTED_EDGE('',*,*,#11483,.T.);
#16887=ORIENTED_EDGE('',*,*,#11484,.T.);
#16888=ORIENTED_EDGE('',*,*,#11485,.T.);
#16889=ORIENTED_EDGE('',*,*,#11486,.T.);
#16890=ORIENTED_EDGE('',*,*,#11487,.T.);
#16891=ORIENTED_EDGE('',*,*,#11485,.F.);
#16892=ORIENTED_EDGE('',*,*,#11488,.T.);
#16893=ORIENTED_EDGE('',*,*,#11475,.T.);
#16894=ORIENTED_EDGE('',*,*,#11489,.T.);
#16895=ORIENTED_EDGE('',*,*,#11472,.F.);
#16896=ORIENTED_EDGE('',*,*,#11490,.T.);
#16897=ORIENTED_EDGE('',*,*,#11467,.F.);
#16898=ORIENTED_EDGE('',*,*,#11469,.F.);
#16899=ORIENTED_EDGE('',*,*,#11491,.T.);
#16900=ORIENTED_EDGE('',*,*,#11492,.T.);
#16901=ORIENTED_EDGE('',*,*,#11493,.T.);
#16902=ORIENTED_EDGE('',*,*,#11494,.T.);
#16903=ORIENTED_EDGE('',*,*,#11468,.F.);
#16904=ORIENTED_EDGE('',*,*,#11495,.F.);
#16905=ORIENTED_EDGE('',*,*,#11496,.F.);
#16906=ORIENTED_EDGE('',*,*,#11491,.F.);
#16907=ORIENTED_EDGE('',*,*,#11471,.F.);
#16908=ORIENTED_EDGE('',*,*,#11479,.F.);
#16909=ORIENTED_EDGE('',*,*,#11488,.F.);
#16910=ORIENTED_EDGE('',*,*,#11497,.F.);
#16911=ORIENTED_EDGE('',*,*,#11490,.F.);
#16912=ORIENTED_EDGE('',*,*,#11497,.T.);
#16913=ORIENTED_EDGE('',*,*,#11487,.F.);
#16914=ORIENTED_EDGE('',*,*,#11495,.T.);
#16915=ORIENTED_EDGE('',*,*,#11483,.F.);
#16916=ORIENTED_EDGE('',*,*,#11498,.T.);
#16917=ORIENTED_EDGE('',*,*,#11499,.T.);
#16918=ORIENTED_EDGE('',*,*,#11500,.T.);
#16919=ORIENTED_EDGE('',*,*,#11501,.F.);
#16920=ORIENTED_EDGE('',*,*,#11492,.F.);
#16921=ORIENTED_EDGE('',*,*,#11502,.F.);
#16922=ORIENTED_EDGE('',*,*,#11486,.F.);
#16923=ORIENTED_EDGE('',*,*,#11503,.T.);
#16924=ORIENTED_EDGE('',*,*,#11502,.T.);
#16925=ORIENTED_EDGE('',*,*,#11496,.T.);
#16926=ORIENTED_EDGE('',*,*,#11484,.F.);
#16927=ORIENTED_EDGE('',*,*,#11504,.T.);
#16928=ORIENTED_EDGE('',*,*,#11501,.T.);
#16929=ORIENTED_EDGE('',*,*,#11505,.T.);
#16930=ORIENTED_EDGE('',*,*,#11481,.F.);
#16931=ORIENTED_EDGE('',*,*,#11505,.F.);
#16932=ORIENTED_EDGE('',*,*,#11503,.F.);
#16933=ORIENTED_EDGE('',*,*,#11489,.F.);
#16934=ORIENTED_EDGE('',*,*,#11466,.F.);
#16935=ORIENTED_EDGE('',*,*,#11506,.T.);
#16936=ORIENTED_EDGE('',*,*,#11507,.T.);
#16937=ORIENTED_EDGE('',*,*,#11473,.F.);
#16938=ORIENTED_EDGE('',*,*,#11508,.F.);
#16939=ORIENTED_EDGE('',*,*,#11509,.T.);
#16940=ORIENTED_EDGE('',*,*,#11510,.T.);
#16941=ORIENTED_EDGE('',*,*,#11511,.T.);
#16942=ORIENTED_EDGE('',*,*,#11512,.T.);
#16943=ORIENTED_EDGE('',*,*,#11513,.F.);
#16944=ORIENTED_EDGE('',*,*,#11514,.T.);
#16945=ORIENTED_EDGE('',*,*,#11515,.T.);
#16946=ORIENTED_EDGE('',*,*,#11516,.T.);
#16947=ORIENTED_EDGE('',*,*,#11517,.T.);
#16948=ORIENTED_EDGE('',*,*,#11516,.F.);
#16949=ORIENTED_EDGE('',*,*,#11518,.T.);
#16950=ORIENTED_EDGE('',*,*,#11519,.T.);
#16951=ORIENTED_EDGE('',*,*,#11520,.T.);
#16952=ORIENTED_EDGE('',*,*,#11521,.T.);
#16953=ORIENTED_EDGE('',*,*,#11522,.T.);
#16954=ORIENTED_EDGE('',*,*,#11523,.T.);
#16955=ORIENTED_EDGE('',*,*,#11524,.T.);
#16956=ORIENTED_EDGE('',*,*,#11525,.T.);
#16957=ORIENTED_EDGE('',*,*,#11526,.T.);
#16958=ORIENTED_EDGE('',*,*,#11523,.F.);
#16959=ORIENTED_EDGE('',*,*,#11525,.F.);
#16960=ORIENTED_EDGE('',*,*,#11527,.T.);
#16961=ORIENTED_EDGE('',*,*,#11514,.F.);
#16962=ORIENTED_EDGE('',*,*,#11521,.F.);
#16963=ORIENTED_EDGE('',*,*,#11528,.T.);
#16964=ORIENTED_EDGE('',*,*,#11510,.F.);
#16965=ORIENTED_EDGE('',*,*,#11512,.F.);
#16966=ORIENTED_EDGE('',*,*,#11529,.T.);
#16967=ORIENTED_EDGE('',*,*,#11530,.T.);
#16968=ORIENTED_EDGE('',*,*,#11531,.T.);
#16969=ORIENTED_EDGE('',*,*,#11532,.T.);
#16970=ORIENTED_EDGE('',*,*,#11511,.F.);
#16971=ORIENTED_EDGE('',*,*,#11533,.F.);
#16972=ORIENTED_EDGE('',*,*,#11534,.F.);
#16973=ORIENTED_EDGE('',*,*,#11529,.F.);
#16974=ORIENTED_EDGE('',*,*,#11519,.F.);
#16975=ORIENTED_EDGE('',*,*,#11533,.T.);
#16976=ORIENTED_EDGE('',*,*,#11528,.F.);
#16977=ORIENTED_EDGE('',*,*,#11535,.T.);
#16978=ORIENTED_EDGE('',*,*,#11536,.F.);
#16979=ORIENTED_EDGE('',*,*,#11537,.F.);
#16980=ORIENTED_EDGE('',*,*,#11538,.F.);
#16981=ORIENTED_EDGE('',*,*,#11539,.T.);
#16982=ORIENTED_EDGE('',*,*,#11540,.T.);
#16983=ORIENTED_EDGE('',*,*,#11537,.T.);
#16984=ORIENTED_EDGE('',*,*,#11541,.T.);
#16985=ORIENTED_EDGE('',*,*,#11542,.F.);
#16986=ORIENTED_EDGE('',*,*,#11530,.F.);
#16987=ORIENTED_EDGE('',*,*,#11543,.F.);
#16988=ORIENTED_EDGE('',*,*,#11518,.F.);
#16989=ORIENTED_EDGE('',*,*,#11544,.T.);
#16990=ORIENTED_EDGE('',*,*,#11543,.T.);
#16991=ORIENTED_EDGE('',*,*,#11534,.T.);
#16992=ORIENTED_EDGE('',*,*,#11542,.T.);
#16993=ORIENTED_EDGE('',*,*,#11545,.T.);
#16994=ORIENTED_EDGE('',*,*,#11538,.T.);
#16995=ORIENTED_EDGE('',*,*,#11546,.T.);
#16996=ORIENTED_EDGE('',*,*,#11527,.F.);
#16997=ORIENTED_EDGE('',*,*,#11547,.T.);
#16998=ORIENTED_EDGE('',*,*,#11536,.T.);
#16999=ORIENTED_EDGE('',*,*,#11548,.T.);
#17000=ORIENTED_EDGE('',*,*,#11515,.F.);
#17001=ORIENTED_EDGE('',*,*,#11548,.F.);
#17002=ORIENTED_EDGE('',*,*,#11545,.F.);
#17003=ORIENTED_EDGE('',*,*,#11544,.F.);
#17004=ORIENTED_EDGE('',*,*,#11509,.F.);
#17005=ORIENTED_EDGE('',*,*,#11549,.T.);
#17006=ORIENTED_EDGE('',*,*,#11550,.T.);
#17007=ORIENTED_EDGE('',*,*,#11551,.T.);
#17008=ORIENTED_EDGE('',*,*,#11522,.F.);
#17009=ORIENTED_EDGE('',*,*,#11552,.T.);
#17010=ORIENTED_EDGE('',*,*,#11553,.T.);
#17011=ORIENTED_EDGE('',*,*,#11554,.T.);
#17012=ORIENTED_EDGE('',*,*,#11555,.T.);
#17013=ORIENTED_EDGE('',*,*,#11554,.F.);
#17014=ORIENTED_EDGE('',*,*,#11556,.T.);
#17015=ORIENTED_EDGE('',*,*,#11557,.T.);
#17016=ORIENTED_EDGE('',*,*,#11552,.F.);
#17017=ORIENTED_EDGE('',*,*,#11558,.T.);
#17018=ORIENTED_EDGE('',*,*,#11559,.T.);
#17019=ORIENTED_EDGE('',*,*,#11559,.F.);
#17020=ORIENTED_EDGE('',*,*,#11560,.T.);
#17021=ORIENTED_EDGE('',*,*,#11561,.F.);
#17022=ORIENTED_EDGE('',*,*,#11562,.T.);
#17023=ORIENTED_EDGE('',*,*,#11558,.F.);
#17024=ORIENTED_EDGE('',*,*,#11563,.T.);
#17025=ORIENTED_EDGE('',*,*,#11564,.T.);
#17026=ORIENTED_EDGE('',*,*,#11565,.T.);
#17027=ORIENTED_EDGE('',*,*,#11555,.F.);
#17028=ORIENTED_EDGE('',*,*,#11566,.F.);
#17029=ORIENTED_EDGE('',*,*,#11567,.F.);
#17030=ORIENTED_EDGE('',*,*,#11563,.F.);
#17031=ORIENTED_EDGE('',*,*,#11568,.F.);
#17032=ORIENTED_EDGE('',*,*,#11569,.T.);
#17033=ORIENTED_EDGE('',*,*,#11570,.T.);
#17034=ORIENTED_EDGE('',*,*,#11571,.T.);
#17035=ORIENTED_EDGE('',*,*,#11572,.T.);
#17036=ORIENTED_EDGE('',*,*,#11573,.F.);
#17037=ORIENTED_EDGE('',*,*,#11574,.T.);
#17038=ORIENTED_EDGE('',*,*,#11575,.T.);
#17039=ORIENTED_EDGE('',*,*,#11576,.T.);
#17040=ORIENTED_EDGE('',*,*,#11577,.T.);
#17041=ORIENTED_EDGE('',*,*,#11578,.T.);
#17042=ORIENTED_EDGE('',*,*,#11579,.T.);
#17043=ORIENTED_EDGE('',*,*,#11580,.T.);
#17044=ORIENTED_EDGE('',*,*,#11581,.T.);
#17045=ORIENTED_EDGE('',*,*,#11582,.T.);
#17046=ORIENTED_EDGE('',*,*,#11583,.T.);
#17047=ORIENTED_EDGE('',*,*,#11580,.F.);
#17048=ORIENTED_EDGE('',*,*,#11584,.T.);
#17049=ORIENTED_EDGE('',*,*,#11576,.F.);
#17050=ORIENTED_EDGE('',*,*,#11574,.F.);
#17051=ORIENTED_EDGE('',*,*,#11561,.T.);
#17052=ORIENTED_EDGE('',*,*,#11570,.F.);
#17053=ORIENTED_EDGE('',*,*,#11572,.F.);
#17054=ORIENTED_EDGE('',*,*,#11585,.T.);
#17055=ORIENTED_EDGE('',*,*,#11586,.F.);
#17056=ORIENTED_EDGE('',*,*,#11587,.T.);
#17057=ORIENTED_EDGE('',*,*,#11588,.T.);
#17058=ORIENTED_EDGE('',*,*,#11571,.F.);
#17059=ORIENTED_EDGE('',*,*,#11560,.F.);
#17060=ORIENTED_EDGE('',*,*,#11565,.F.);
#17061=ORIENTED_EDGE('',*,*,#11585,.F.);
#17062=ORIENTED_EDGE('',*,*,#11553,.F.);
#17063=ORIENTED_EDGE('',*,*,#11562,.F.);
#17064=ORIENTED_EDGE('',*,*,#11577,.F.);
#17065=ORIENTED_EDGE('',*,*,#11589,.F.);
#17066=ORIENTED_EDGE('',*,*,#11556,.F.);
#17067=ORIENTED_EDGE('',*,*,#11589,.T.);
#17068=ORIENTED_EDGE('',*,*,#11584,.F.);
#17069=ORIENTED_EDGE('',*,*,#11590,.T.);
#17070=ORIENTED_EDGE('',*,*,#11579,.F.);
#17071=ORIENTED_EDGE('',*,*,#11591,.F.);
#17072=ORIENTED_EDGE('',*,*,#11592,.F.);
#17073=ORIENTED_EDGE('',*,*,#11590,.F.);
#17074=ORIENTED_EDGE('',*,*,#11578,.F.);
#17075=ORIENTED_EDGE('',*,*,#11593,.T.);
#17076=ORIENTED_EDGE('',*,*,#11594,.T.);
#17077=ORIENTED_EDGE('',*,*,#11595,.T.);
#17078=ORIENTED_EDGE('',*,*,#11591,.T.);
#17079=ORIENTED_EDGE('',*,*,#11596,.F.);
#17080=ORIENTED_EDGE('',*,*,#11550,.F.);
#17081=ORIENTED_EDGE('',*,*,#11597,.T.);
#17082=ORIENTED_EDGE('',*,*,#11598,.T.);
#17083=ORIENTED_EDGE('',*,*,#11599,.T.);
#17084=ORIENTED_EDGE('',*,*,#11597,.F.);
#17085=ORIENTED_EDGE('',*,*,#11549,.F.);
#17086=ORIENTED_EDGE('',*,*,#11508,.T.);
#17087=ORIENTED_EDGE('',*,*,#11600,.F.);
#17088=ORIENTED_EDGE('',*,*,#11582,.F.);
#17089=ORIENTED_EDGE('',*,*,#11601,.T.);
#17090=ORIENTED_EDGE('',*,*,#11568,.T.);
#17091=ORIENTED_EDGE('',*,*,#11602,.F.);
#17092=ORIENTED_EDGE('',*,*,#11603,.T.);
#17093=ORIENTED_EDGE('',*,*,#11604,.T.);
#17094=ORIENTED_EDGE('',*,*,#11605,.F.);
#17095=ORIENTED_EDGE('',*,*,#11606,.T.);
#17096=ORIENTED_EDGE('',*,*,#11607,.F.);
#17097=ORIENTED_EDGE('',*,*,#11506,.F.);
#17098=ORIENTED_EDGE('',*,*,#11465,.T.);
#17099=ORIENTED_EDGE('',*,*,#11608,.F.);
#17100=ORIENTED_EDGE('',*,*,#11606,.F.);
#17101=ORIENTED_EDGE('',*,*,#11609,.T.);
#17102=ORIENTED_EDGE('',*,*,#11610,.F.);
#17103=ORIENTED_EDGE('',*,*,#11611,.T.);
#17104=ORIENTED_EDGE('',*,*,#11612,.F.);
#17105=ORIENTED_EDGE('',*,*,#11613,.F.);
#17106=ORIENTED_EDGE('',*,*,#11602,.T.);
#17107=ORIENTED_EDGE('',*,*,#11573,.T.);
#17108=ORIENTED_EDGE('',*,*,#11588,.F.);
#17109=ORIENTED_EDGE('',*,*,#11614,.T.);
#17110=ORIENTED_EDGE('',*,*,#11593,.F.);
#17111=ORIENTED_EDGE('',*,*,#11583,.F.);
#17112=ORIENTED_EDGE('',*,*,#11600,.T.);
#17113=ORIENTED_EDGE('',*,*,#11513,.T.);
#17114=ORIENTED_EDGE('',*,*,#11532,.F.);
#17115=ORIENTED_EDGE('',*,*,#11615,.T.);
#17116=ORIENTED_EDGE('',*,*,#11539,.F.);
#17117=ORIENTED_EDGE('',*,*,#11616,.T.);
#17118=ORIENTED_EDGE('',*,*,#11608,.T.);
#17119=ORIENTED_EDGE('',*,*,#11470,.T.);
#17120=ORIENTED_EDGE('',*,*,#11494,.F.);
#17121=ORIENTED_EDGE('',*,*,#11617,.T.);
#17122=ORIENTED_EDGE('',*,*,#11499,.F.);
#17123=ORIENTED_EDGE('',*,*,#11618,.T.);
#17124=ORIENTED_EDGE('',*,*,#11619,.F.);
#17125=ORIENTED_EDGE('',*,*,#11598,.F.);
#17126=ORIENTED_EDGE('',*,*,#11599,.F.);
#17127=ORIENTED_EDGE('',*,*,#11620,.T.);
#17128=ORIENTED_EDGE('',*,*,#11621,.F.);
#17129=ORIENTED_EDGE('',*,*,#11622,.F.);
#17130=ORIENTED_EDGE('',*,*,#11620,.F.);
#17131=ORIENTED_EDGE('',*,*,#11623,.T.);
#17132=ORIENTED_EDGE('',*,*,#11624,.T.);
#17133=ORIENTED_EDGE('',*,*,#11625,.T.);
#17134=ORIENTED_EDGE('',*,*,#11626,.T.);
#17135=ORIENTED_EDGE('',*,*,#11624,.F.);
#17136=ORIENTED_EDGE('',*,*,#11626,.F.);
#17137=ORIENTED_EDGE('',*,*,#11627,.T.);
#17138=ORIENTED_EDGE('',*,*,#11628,.F.);
#17139=ORIENTED_EDGE('',*,*,#11629,.F.);
#17140=ORIENTED_EDGE('',*,*,#11627,.F.);
#17141=ORIENTED_EDGE('',*,*,#11625,.F.);
#17142=ORIENTED_EDGE('',*,*,#11623,.F.);
#17143=ORIENTED_EDGE('',*,*,#11630,.F.);
#17144=ORIENTED_EDGE('',*,*,#11631,.F.);
#17145=ORIENTED_EDGE('',*,*,#11595,.F.);
#17146=ORIENTED_EDGE('',*,*,#11632,.F.);
#17147=ORIENTED_EDGE('',*,*,#11633,.T.);
#17148=ORIENTED_EDGE('',*,*,#11567,.T.);
#17149=ORIENTED_EDGE('',*,*,#11632,.T.);
#17150=ORIENTED_EDGE('',*,*,#11634,.T.);
#17151=ORIENTED_EDGE('',*,*,#11557,.F.);
#17152=ORIENTED_EDGE('',*,*,#11592,.T.);
#17153=ORIENTED_EDGE('',*,*,#11631,.T.);
#17154=ORIENTED_EDGE('',*,*,#11566,.T.);
#17155=ORIENTED_EDGE('',*,*,#11633,.F.);
#17156=ORIENTED_EDGE('',*,*,#11586,.T.);
#17157=ORIENTED_EDGE('',*,*,#11564,.F.);
#17158=ORIENTED_EDGE('',*,*,#11569,.F.);
#17159=ORIENTED_EDGE('',*,*,#11601,.F.);
#17160=ORIENTED_EDGE('',*,*,#11581,.F.);
#17161=ORIENTED_EDGE('',*,*,#11575,.F.);
#17162=ORIENTED_EDGE('',*,*,#11634,.F.);
#17163=ORIENTED_EDGE('',*,*,#11594,.F.);
#17164=ORIENTED_EDGE('',*,*,#11614,.F.);
#17165=ORIENTED_EDGE('',*,*,#11587,.F.);
#17166=ORIENTED_EDGE('',*,*,#11635,.T.);
#17167=ORIENTED_EDGE('',*,*,#11636,.T.);
#17168=ORIENTED_EDGE('',*,*,#11637,.T.);
#17169=ORIENTED_EDGE('',*,*,#11638,.T.);
#17170=ORIENTED_EDGE('',*,*,#11603,.F.);
#17171=ORIENTED_EDGE('',*,*,#11613,.T.);
#17172=ORIENTED_EDGE('',*,*,#11639,.T.);
#17173=ORIENTED_EDGE('',*,*,#11640,.T.);
#17174=ORIENTED_EDGE('',*,*,#11641,.T.);
#17175=ORIENTED_EDGE('',*,*,#11642,.T.);
#17176=ORIENTED_EDGE('',*,*,#11643,.T.);
#17177=ORIENTED_EDGE('',*,*,#11644,.T.);
#17178=ORIENTED_EDGE('',*,*,#11645,.T.);
#17179=ORIENTED_EDGE('',*,*,#11646,.T.);
#17180=ORIENTED_EDGE('',*,*,#11645,.F.);
#17181=ORIENTED_EDGE('',*,*,#11647,.T.);
#17182=ORIENTED_EDGE('',*,*,#11648,.T.);
#17183=ORIENTED_EDGE('',*,*,#11643,.F.);
#17184=ORIENTED_EDGE('',*,*,#11649,.T.);
#17185=ORIENTED_EDGE('',*,*,#11641,.F.);
#17186=ORIENTED_EDGE('',*,*,#11639,.F.);
#17187=ORIENTED_EDGE('',*,*,#11650,.T.);
#17188=ORIENTED_EDGE('',*,*,#11637,.F.);
#17189=ORIENTED_EDGE('',*,*,#11638,.F.);
#17190=ORIENTED_EDGE('',*,*,#11651,.F.);
#17191=ORIENTED_EDGE('',*,*,#11652,.F.);
#17192=ORIENTED_EDGE('',*,*,#11604,.F.);
#17193=ORIENTED_EDGE('',*,*,#11650,.F.);
#17194=ORIENTED_EDGE('',*,*,#11653,.T.);
#17195=ORIENTED_EDGE('',*,*,#11654,.T.);
#17196=ORIENTED_EDGE('',*,*,#11651,.T.);
#17197=ORIENTED_EDGE('',*,*,#11642,.F.);
#17198=ORIENTED_EDGE('',*,*,#11655,.F.);
#17199=ORIENTED_EDGE('',*,*,#11656,.F.);
#17200=ORIENTED_EDGE('',*,*,#11653,.F.);
#17201=ORIENTED_EDGE('',*,*,#11649,.F.);
#17202=ORIENTED_EDGE('',*,*,#11657,.T.);
#17203=ORIENTED_EDGE('',*,*,#11658,.F.);
#17204=ORIENTED_EDGE('',*,*,#11655,.T.);
#17205=ORIENTED_EDGE('',*,*,#11646,.F.);
#17206=ORIENTED_EDGE('',*,*,#11659,.F.);
#17207=ORIENTED_EDGE('',*,*,#11660,.F.);
#17208=ORIENTED_EDGE('',*,*,#11657,.F.);
#17209=ORIENTED_EDGE('',*,*,#11628,.T.);
#17210=ORIENTED_EDGE('',*,*,#11629,.T.);
#17211=ORIENTED_EDGE('',*,*,#11661,.T.);
#17212=ORIENTED_EDGE('',*,*,#11662,.T.);
#17213=ORIENTED_EDGE('',*,*,#11663,.T.);
#17214=ORIENTED_EDGE('',*,*,#11661,.F.);
#17215=ORIENTED_EDGE('',*,*,#11663,.F.);
#17216=ORIENTED_EDGE('',*,*,#11664,.T.);
#17217=ORIENTED_EDGE('',*,*,#11665,.F.);
#17218=ORIENTED_EDGE('',*,*,#11666,.F.);
#17219=ORIENTED_EDGE('',*,*,#11664,.F.);
#17220=ORIENTED_EDGE('',*,*,#11662,.F.);
#17221=ORIENTED_EDGE('',*,*,#11621,.T.);
#17222=ORIENTED_EDGE('',*,*,#11622,.T.);
#17223=ORIENTED_EDGE('',*,*,#11667,.T.);
#17224=ORIENTED_EDGE('',*,*,#11668,.T.);
#17225=ORIENTED_EDGE('',*,*,#11669,.T.);
#17226=ORIENTED_EDGE('',*,*,#11667,.F.);
#17227=ORIENTED_EDGE('',*,*,#11669,.F.);
#17228=ORIENTED_EDGE('',*,*,#11670,.T.);
#17229=ORIENTED_EDGE('',*,*,#11630,.T.);
#17230=ORIENTED_EDGE('',*,*,#11670,.F.);
#17231=ORIENTED_EDGE('',*,*,#11668,.F.);
#17232=ORIENTED_EDGE('',*,*,#11671,.F.);
#17233=ORIENTED_EDGE('',*,*,#11672,.T.);
#17234=ORIENTED_EDGE('',*,*,#11619,.T.);
#17235=ORIENTED_EDGE('',*,*,#11672,.F.);
#17236=ORIENTED_EDGE('',*,*,#11665,.T.);
#17237=ORIENTED_EDGE('',*,*,#11666,.T.);
#17238=ORIENTED_EDGE('',*,*,#11673,.T.);
#17239=ORIENTED_EDGE('',*,*,#11674,.T.);
#17240=ORIENTED_EDGE('',*,*,#11673,.F.);
#17241=ORIENTED_EDGE('',*,*,#11674,.F.);
#17242=ORIENTED_EDGE('',*,*,#11675,.F.);
#17243=ORIENTED_EDGE('',*,*,#11652,.T.);
#17244=ORIENTED_EDGE('',*,*,#11676,.T.);
#17245=ORIENTED_EDGE('',*,*,#11677,.T.);
#17246=ORIENTED_EDGE('',*,*,#11678,.T.);
#17247=ORIENTED_EDGE('',*,*,#11609,.F.);
#17248=ORIENTED_EDGE('',*,*,#11605,.T.);
#17249=ORIENTED_EDGE('',*,*,#11654,.F.);
#17250=ORIENTED_EDGE('',*,*,#11679,.T.);
#17251=ORIENTED_EDGE('',*,*,#11676,.F.);
#17252=ORIENTED_EDGE('',*,*,#11678,.F.);
#17253=ORIENTED_EDGE('',*,*,#11680,.T.);
#17254=ORIENTED_EDGE('',*,*,#11681,.T.);
#17255=ORIENTED_EDGE('',*,*,#11682,.T.);
#17256=ORIENTED_EDGE('',*,*,#11610,.T.);
#17257=ORIENTED_EDGE('',*,*,#11677,.F.);
#17258=ORIENTED_EDGE('',*,*,#11683,.F.);
#17259=ORIENTED_EDGE('',*,*,#11684,.F.);
#17260=ORIENTED_EDGE('',*,*,#11680,.F.);
#17261=ORIENTED_EDGE('',*,*,#11679,.F.);
#17262=ORIENTED_EDGE('',*,*,#11656,.T.);
#17263=ORIENTED_EDGE('',*,*,#11685,.F.);
#17264=ORIENTED_EDGE('',*,*,#11683,.T.);
#17265=ORIENTED_EDGE('',*,*,#11636,.F.);
#17266=ORIENTED_EDGE('',*,*,#11686,.F.);
#17267=ORIENTED_EDGE('',*,*,#11644,.F.);
#17268=ORIENTED_EDGE('',*,*,#11640,.F.);
#17269=ORIENTED_EDGE('',*,*,#11658,.T.);
#17270=ORIENTED_EDGE('',*,*,#11687,.T.);
#17271=ORIENTED_EDGE('',*,*,#11685,.T.);
#17272=ORIENTED_EDGE('',*,*,#11635,.F.);
#17273=ORIENTED_EDGE('',*,*,#11612,.T.);
#17274=ORIENTED_EDGE('',*,*,#11688,.T.);
#17275=ORIENTED_EDGE('',*,*,#11647,.F.);
#17276=ORIENTED_EDGE('',*,*,#11686,.T.);
#17277=ORIENTED_EDGE('',*,*,#11689,.F.);
#17278=ORIENTED_EDGE('',*,*,#11681,.F.);
#17279=ORIENTED_EDGE('',*,*,#11690,.F.);
#17280=ORIENTED_EDGE('',*,*,#11687,.F.);
#17281=ORIENTED_EDGE('',*,*,#11660,.T.);
#17282=ORIENTED_EDGE('',*,*,#11690,.T.);
#17283=ORIENTED_EDGE('',*,*,#11684,.T.);
#17284=ORIENTED_EDGE('',*,*,#11648,.F.);
#17285=ORIENTED_EDGE('',*,*,#11691,.T.);
#17286=ORIENTED_EDGE('',*,*,#11689,.T.);
#17287=ORIENTED_EDGE('',*,*,#11659,.T.);
#17288=ORIENTED_EDGE('',*,*,#11675,.T.);
#17289=ORIENTED_EDGE('',*,*,#11692,.T.);
#17290=ORIENTED_EDGE('',*,*,#11693,.T.);
#17291=ORIENTED_EDGE('',*,*,#11694,.T.);
#17292=ORIENTED_EDGE('',*,*,#11692,.F.);
#17293=ORIENTED_EDGE('',*,*,#11695,.F.);
#17294=ORIENTED_EDGE('',*,*,#11696,.T.);
#17295=ORIENTED_EDGE('',*,*,#11693,.F.);
#17296=ORIENTED_EDGE('',*,*,#11694,.F.);
#17297=ORIENTED_EDGE('',*,*,#11696,.F.);
#17298=ORIENTED_EDGE('',*,*,#11697,.F.);
#17299=ORIENTED_EDGE('',*,*,#11695,.T.);
#17300=ORIENTED_EDGE('',*,*,#11698,.T.);
#17301=ORIENTED_EDGE('',*,*,#11699,.T.);
#17302=ORIENTED_EDGE('',*,*,#11698,.F.);
#17303=ORIENTED_EDGE('',*,*,#11697,.T.);
#17304=ORIENTED_EDGE('',*,*,#11700,.T.);
#17305=ORIENTED_EDGE('',*,*,#11699,.F.);
#17306=ORIENTED_EDGE('',*,*,#11700,.F.);
#17307=ORIENTED_EDGE('',*,*,#11701,.T.);
#17308=ORIENTED_EDGE('',*,*,#11671,.T.);
#17309=ORIENTED_EDGE('',*,*,#11701,.F.);
#17310=ORIENTED_EDGE('',*,*,#11688,.F.);
#17311=ORIENTED_EDGE('',*,*,#11611,.F.);
#17312=ORIENTED_EDGE('',*,*,#11682,.F.);
#17313=ORIENTED_EDGE('',*,*,#11691,.F.);
#17314=ORIENTED_EDGE('',*,*,#11540,.F.);
#17315=ORIENTED_EDGE('',*,*,#11615,.F.);
#17316=ORIENTED_EDGE('',*,*,#11531,.F.);
#17317=ORIENTED_EDGE('',*,*,#11546,.F.);
#17318=ORIENTED_EDGE('',*,*,#11524,.F.);
#17319=ORIENTED_EDGE('',*,*,#11551,.F.);
#17320=ORIENTED_EDGE('',*,*,#11596,.T.);
#17321=ORIENTED_EDGE('',*,*,#11616,.F.);
#17322=ORIENTED_EDGE('',*,*,#11541,.F.);
#17323=ORIENTED_EDGE('',*,*,#11547,.F.);
#17324=ORIENTED_EDGE('',*,*,#11517,.F.);
#17325=ORIENTED_EDGE('',*,*,#11535,.F.);
#17326=ORIENTED_EDGE('',*,*,#11520,.F.);
#17327=ORIENTED_EDGE('',*,*,#11526,.F.);
#17328=ORIENTED_EDGE('',*,*,#11500,.F.);
#17329=ORIENTED_EDGE('',*,*,#11617,.F.);
#17330=ORIENTED_EDGE('',*,*,#11493,.F.);
#17331=ORIENTED_EDGE('',*,*,#11504,.F.);
#17332=ORIENTED_EDGE('',*,*,#11478,.F.);
#17333=ORIENTED_EDGE('',*,*,#11507,.F.);
#17334=ORIENTED_EDGE('',*,*,#11607,.T.);
#17335=ORIENTED_EDGE('',*,*,#11618,.F.);
#17336=ORIENTED_EDGE('',*,*,#11498,.F.);
#17337=ORIENTED_EDGE('',*,*,#11482,.F.);
#18725=CYLINDRICAL_SURFACE('',#21778,0.4);
#18726=CYLINDRICAL_SURFACE('',#21781,0.4);
#18727=CYLINDRICAL_SURFACE('',#21788,0.4);
#18728=CYLINDRICAL_SURFACE('',#21789,0.4);
#18729=CYLINDRICAL_SURFACE('',#21798,0.4);
#18730=CYLINDRICAL_SURFACE('',#21801,0.4);
#18731=CYLINDRICAL_SURFACE('',#21806,0.4);
#18732=CYLINDRICAL_SURFACE('',#21807,0.4);
#18733=CYLINDRICAL_SURFACE('',#21812,0.4);
#18734=CYLINDRICAL_SURFACE('',#21813,0.4);
#18735=CYLINDRICAL_SURFACE('',#21817,0.4);
#18736=CYLINDRICAL_SURFACE('',#21820,0.4);
#18737=CYLINDRICAL_SURFACE('',#21826,0.4);
#18738=CYLINDRICAL_SURFACE('',#21829,0.4);
#18739=CYLINDRICAL_SURFACE('',#21835,0.4);
#18740=CYLINDRICAL_SURFACE('',#21839,0.4);
#18741=CYLINDRICAL_SURFACE('',#21844,0.4);
#18742=CYLINDRICAL_SURFACE('',#21849,0.4);
#18743=CYLINDRICAL_SURFACE('',#21850,0.4);
#18744=CYLINDRICAL_SURFACE('',#21851,0.4);
#18745=CYLINDRICAL_SURFACE('',#21856,0.4);
#18746=CYLINDRICAL_SURFACE('',#21865,0.4);
#18747=CYLINDRICAL_SURFACE('',#21867,0.4);
#18748=CYLINDRICAL_SURFACE('',#21870,0.4);
#18749=CYLINDRICAL_SURFACE('',#21873,0.4);
#18750=CYLINDRICAL_SURFACE('',#21876,0.4);
#18751=CYLINDRICAL_SURFACE('',#21882,0.4);
#18752=CYLINDRICAL_SURFACE('',#21887,0.4);
#18753=CYLINDRICAL_SURFACE('',#21889,0.4);
#18754=CYLINDRICAL_SURFACE('',#21914,23.);
#18755=CYLINDRICAL_SURFACE('',#21922,0.4);
#18756=CYLINDRICAL_SURFACE('',#21924,0.4);
#18757=CYLINDRICAL_SURFACE('',#21928,0.4);
#18758=CYLINDRICAL_SURFACE('',#21931,0.4);
#18759=CYLINDRICAL_SURFACE('',#21934,0.4);
#18760=CYLINDRICAL_SURFACE('',#21945,0.4);
#18761=CYLINDRICAL_SURFACE('',#21948,0.4);
#18762=CYLINDRICAL_SURFACE('',#21962,21.8);
#18763=CYLINDRICAL_SURFACE('',#21971,0.4);
#18764=CYLINDRICAL_SURFACE('',#21976,0.4);
#18765=CYLINDRICAL_SURFACE('',#21979,0.4);
#18766=CYLINDRICAL_SURFACE('',#21984,0.4);
#18767=CYLINDRICAL_SURFACE('',#21988,0.4);
#18768=CYLINDRICAL_SURFACE('',#21989,0.4);
#18769=CYLINDRICAL_SURFACE('',#21994,7.05);
#18770=CYLINDRICAL_SURFACE('',#22002,10.4);
#19712=ADVANCED_FACE('',(#2016),#18725,.T.);
#19713=ADVANCED_FACE('',(#2017),#18726,.T.);
#19714=ADVANCED_FACE('',(#2018),#292,.T.);
#19715=ADVANCED_FACE('',(#2019),#18727,.T.);
#19716=ADVANCED_FACE('',(#2020),#18728,.T.);
#19717=ADVANCED_FACE('',(#2021),#293,.T.);
#19718=ADVANCED_FACE('',(#2022),#294,.T.);
#19719=ADVANCED_FACE('',(#2023),#18729,.T.);
#19720=ADVANCED_FACE('',(#2024),#295,.T.);
#19721=ADVANCED_FACE('',(#2025),#18730,.T.);
#19722=ADVANCED_FACE('',(#2026),#984,.T.);
#19723=ADVANCED_FACE('',(#2027),#985,.T.);
#19724=ADVANCED_FACE('',(#2028),#18731,.T.);
#19725=ADVANCED_FACE('',(#2029),#18732,.T.);
#19726=ADVANCED_FACE('',(#2030),#296,.T.);
#19727=ADVANCED_FACE('',(#2031),#18733,.T.);
#19728=ADVANCED_FACE('',(#2032),#18734,.T.);
#19729=ADVANCED_FACE('',(#2033),#986,.T.);
#19730=ADVANCED_FACE('',(#2034),#987,.F.);
#19731=ADVANCED_FACE('',(#2035),#18735,.T.);
#19732=ADVANCED_FACE('',(#2036),#18736,.T.);
#19733=ADVANCED_FACE('',(#2037),#297,.T.);
#19734=ADVANCED_FACE('',(#2038),#18737,.T.);
#19735=ADVANCED_FACE('',(#2039),#18738,.T.);
#19736=ADVANCED_FACE('',(#2040),#298,.T.);
#19737=ADVANCED_FACE('',(#2041),#299,.T.);
#19738=ADVANCED_FACE('',(#2042),#18739,.T.);
#19739=ADVANCED_FACE('',(#2043),#988,.T.);
#19740=ADVANCED_FACE('',(#2044),#18740,.T.);
#19741=ADVANCED_FACE('',(#2045),#300,.T.);
#19742=ADVANCED_FACE('',(#2046),#18741,.T.);
#19743=ADVANCED_FACE('',(#2047),#301,.T.);
#19744=ADVANCED_FACE('',(#2048),#18742,.T.);
#19745=ADVANCED_FACE('',(#2049),#18743,.T.);
#19746=ADVANCED_FACE('',(#2050),#18744,.T.);
#19747=ADVANCED_FACE('',(#2051),#989,.T.);
#19748=ADVANCED_FACE('',(#2052),#990,.F.);
#19749=ADVANCED_FACE('',(#2053),#18745,.T.);
#19750=ADVANCED_FACE('',(#2054),#302,.T.);
#19751=ADVANCED_FACE('',(#2055),#303,.T.);
#19752=ADVANCED_FACE('',(#2056),#18746,.T.);
#19753=ADVANCED_FACE('',(#2057),#18747,.T.);
#19754=ADVANCED_FACE('',(#2058),#991,.T.);
#19755=ADVANCED_FACE('',(#2059),#18748,.T.);
#19756=ADVANCED_FACE('',(#2060),#18749,.T.);
#19757=ADVANCED_FACE('',(#2061),#18750,.T.);
#19758=ADVANCED_FACE('',(#2062),#304,.T.);
#19759=ADVANCED_FACE('',(#2063),#305,.T.);
#19760=ADVANCED_FACE('',(#2064),#18751,.T.);
#19761=ADVANCED_FACE('',(#2065),#992,.T.);
#19762=ADVANCED_FACE('',(#2066),#993,.T.);
#19763=ADVANCED_FACE('',(#2067),#18752,.T.);
#19764=ADVANCED_FACE('',(#2068),#994,.T.);
#19765=ADVANCED_FACE('',(#2069),#18753,.T.);
#19766=ADVANCED_FACE('',(#2070),#160,.T.);
#19767=ADVANCED_FACE('',(#2071,#1120),#995,.T.);
#19768=ADVANCED_FACE('',(#2072),#493,.T.);
#19769=ADVANCED_FACE('',(#2073),#161,.T.);
#19770=ADVANCED_FACE('',(#2074),#18754,.T.);
#19771=ADVANCED_FACE('',(#2075,#1121),#996,.T.);
#19772=ADVANCED_FACE('',(#2076),#306,.T.);
#19773=ADVANCED_FACE('',(#2077),#18755,.T.);
#19774=ADVANCED_FACE('',(#2078),#18756,.T.);
#19775=ADVANCED_FACE('',(#2079),#307,.T.);
#19776=ADVANCED_FACE('',(#2080),#997,.F.);
#19777=ADVANCED_FACE('',(#2081),#998,.T.);
#19778=ADVANCED_FACE('',(#2082),#18757,.T.);
#19779=ADVANCED_FACE('',(#2083),#18758,.T.);
#19780=ADVANCED_FACE('',(#2084),#18759,.T.);
#19781=ADVANCED_FACE('',(#2085),#308,.T.);
#19782=ADVANCED_FACE('',(#2086),#309,.T.);
#19783=ADVANCED_FACE('',(#2087),#310,.T.);
#19784=ADVANCED_FACE('',(#2088),#999,.F.);
#19785=ADVANCED_FACE('',(#2089),#18760,.T.);
#19786=ADVANCED_FACE('',(#2090),#1000,.T.);
#19787=ADVANCED_FACE('',(#2091),#18761,.T.);
#19788=ADVANCED_FACE('',(#2092),#1001,.T.);
#19789=ADVANCED_FACE('',(#2093),#162,.T.);
#19790=ADVANCED_FACE('',(#2094),#494,.T.);
#19791=ADVANCED_FACE('',(#2095),#163,.T.);
#19792=ADVANCED_FACE('',(#2096),#18762,.T.);
#19793=ADVANCED_FACE('',(#2097),#164,.T.);
#19794=ADVANCED_FACE('',(#2098),#165,.T.);
#19795=ADVANCED_FACE('',(#2099,#1122),#1002,.T.);
#19796=ADVANCED_FACE('',(#2100),#18763,.T.);
#19797=ADVANCED_FACE('',(#2101),#311,.T.);
#19798=ADVANCED_FACE('',(#2102),#18764,.T.);
#19799=ADVANCED_FACE('',(#2103),#1003,.T.);
#19800=ADVANCED_FACE('',(#2104),#18765,.T.);
#19801=ADVANCED_FACE('',(#2105),#1004,.T.);
#19802=ADVANCED_FACE('',(#2106),#312,.T.);
#19803=ADVANCED_FACE('',(#2107),#18766,.T.);
#19804=ADVANCED_FACE('',(#2108),#313,.T.);
#19805=ADVANCED_FACE('',(#2109),#18767,.T.);
#19806=ADVANCED_FACE('',(#2110),#18768,.T.);
#19807=ADVANCED_FACE('',(#2111),#166,.T.);
#19808=ADVANCED_FACE('',(#2112),#18769,.F.);
#19809=ADVANCED_FACE('',(#2113),#167,.T.);
#19810=ADVANCED_FACE('',(#2114,#1123),#1005,.F.);
#19811=ADVANCED_FACE('',(#2115),#18770,.F.);
#19812=ADVANCED_FACE('',(#2116),#1006,.T.);
#19813=ADVANCED_FACE('',(#2117),#1007,.T.);
#19814=ADVANCED_FACE('',(#2118),#1008,.T.);
#19815=ADVANCED_FACE('',(#2119),#1009,.T.);
#19816=ADVANCED_FACE('',(#2120),#1010,.T.);
#19817=ADVANCED_FACE('',(#2121),#1011,.T.);
#20015=CLOSED_SHELL('',(#19712,#19713,#19714,#19715,#19716,#19717,#19718,
#19719,#19720,#19721,#19722,#19723,#19724,#19725,#19726,#19727,#19728,#19729,
#19730,#19731,#19732,#19733,#19734,#19735,#19736,#19737,#19738,#19739,#19740,
#19741,#19742,#19743,#19744,#19745,#19746,#19747,#19748,#19749,#19750,#19751,
#19752,#19753,#19754,#19755,#19756,#19757,#19758,#19759,#19760,#19761,#19762,
#19763,#19764,#19765,#19766,#19767,#19768,#19769,#19770,#19771,#19772,#19773,
#19774,#19775,#19776,#19777,#19778,#19779,#19780,#19781,#19782,#19783,#19784,
#19785,#19786,#19787,#19788,#19789,#19790,#19791,#19792,#19793,#19794,#19795,
#19796,#19797,#19798,#19799,#19800,#19801,#19802,#19803,#19804,#19805,#19806,
#19807,#19808,#19809,#19810,#19811,#19812,#19813,#19814,#19815,#19816,#19817));
#21777=AXIS2_PLACEMENT_3D('',#62000,#26259,#26260);
#21778=AXIS2_PLACEMENT_3D('',#62001,#26261,#26262);
#21779=AXIS2_PLACEMENT_3D('',#62022,#26264,#26265);
#21780=AXIS2_PLACEMENT_3D('',#62026,#26267,#26268);
#21781=AXIS2_PLACEMENT_3D('',#62028,#26270,#26271);
#21782=AXIS2_PLACEMENT_3D('',#62032,#26273,#26274);
#21783=AXIS2_PLACEMENT_3D('',#62035,#26276,#26277);
#21784=AXIS2_PLACEMENT_3D('',#62036,#26278,#26279);
#21785=AXIS2_PLACEMENT_3D('',#62039,#26280,#26281);
#21786=AXIS2_PLACEMENT_3D('',#62041,#26282,#26283);
#21787=AXIS2_PLACEMENT_3D('',#62042,#26284,#26285);
#21788=AXIS2_PLACEMENT_3D('',#62043,#26286,#26287);
#21789=AXIS2_PLACEMENT_3D('',#62046,#26290,#26291);
#21790=AXIS2_PLACEMENT_3D('',#62049,#26292,#26293);
#21791=AXIS2_PLACEMENT_3D('',#62052,#26296,#26297);
#21792=AXIS2_PLACEMENT_3D('',#62054,#26298,#26299);
#21793=AXIS2_PLACEMENT_3D('',#62055,#26300,#26301);
#21794=AXIS2_PLACEMENT_3D('',#62056,#26302,#26303);
#21795=AXIS2_PLACEMENT_3D('',#62059,#26304,#26305);
#21796=AXIS2_PLACEMENT_3D('',#62061,#26306,#26307);
#21797=AXIS2_PLACEMENT_3D('',#62062,#26308,#26309);
#21798=AXIS2_PLACEMENT_3D('',#62063,#26310,#26311);
#21799=AXIS2_PLACEMENT_3D('',#62066,#26314,#26315);
#21800=AXIS2_PLACEMENT_3D('',#62067,#26316,#26317);
#21801=AXIS2_PLACEMENT_3D('',#62068,#26318,#26319);
#21802=AXIS2_PLACEMENT_3D('',#62072,#26321,#26322);
#21803=AXIS2_PLACEMENT_3D('',#62075,#26324,#26325);
#21804=AXIS2_PLACEMENT_3D('',#62076,#26326,#26327);
#21805=AXIS2_PLACEMENT_3D('',#62079,#26330,#26331);
#21806=AXIS2_PLACEMENT_3D('',#62081,#26333,#26334);
#21807=AXIS2_PLACEMENT_3D('',#62082,#26335,#26336);
#21808=AXIS2_PLACEMENT_3D('',#62086,#26338,#26339);
#21809=AXIS2_PLACEMENT_3D('',#62088,#26341,#26342);
#21810=AXIS2_PLACEMENT_3D('',#62090,#26343,#26344);
#21811=AXIS2_PLACEMENT_3D('',#62091,#26345,#26346);
#21812=AXIS2_PLACEMENT_3D('',#62092,#26347,#26348);
#21813=AXIS2_PLACEMENT_3D('',#62094,#26350,#26351);
#21814=AXIS2_PLACEMENT_3D('',#62097,#26354,#26355);
#21815=AXIS2_PLACEMENT_3D('',#62098,#26356,#26357);
#21816=AXIS2_PLACEMENT_3D('',#62100,#26358,#26359);
#21817=AXIS2_PLACEMENT_3D('',#62102,#26361,#26362);
#21818=AXIS2_PLACEMENT_3D('',#62123,#26364,#26365);
#21819=AXIS2_PLACEMENT_3D('',#62127,#26367,#26368);
#21820=AXIS2_PLACEMENT_3D('',#62129,#26370,#26371);
#21821=AXIS2_PLACEMENT_3D('',#62132,#26372,#26373);
#21822=AXIS2_PLACEMENT_3D('',#62136,#26375,#26376);
#21823=AXIS2_PLACEMENT_3D('',#62138,#26378,#26379);
#21824=AXIS2_PLACEMENT_3D('',#62140,#26380,#26381);
#21825=AXIS2_PLACEMENT_3D('',#62141,#26382,#26383);
#21826=AXIS2_PLACEMENT_3D('',#62142,#26384,#26385);
#21827=AXIS2_PLACEMENT_3D('',#62146,#26387,#26388);
#21828=AXIS2_PLACEMENT_3D('',#62149,#26390,#26391);
#21829=AXIS2_PLACEMENT_3D('',#62150,#26392,#26393);
#21830=AXIS2_PLACEMENT_3D('',#62153,#26395,#26396);
#21831=AXIS2_PLACEMENT_3D('',#62155,#26398,#26399);
#21832=AXIS2_PLACEMENT_3D('',#62156,#26400,#26401);
#21833=AXIS2_PLACEMENT_3D('',#62157,#26402,#26403);
#21834=AXIS2_PLACEMENT_3D('',#62158,#26404,#26405);
#21835=AXIS2_PLACEMENT_3D('',#62159,#26406,#26407);
#21836=AXIS2_PLACEMENT_3D('',#62163,#26409,#26410);
#21837=AXIS2_PLACEMENT_3D('',#62166,#26412,#26413);
#21838=AXIS2_PLACEMENT_3D('',#62167,#26414,#26415);
#21839=AXIS2_PLACEMENT_3D('',#62170,#26418,#26419);
#21840=AXIS2_PLACEMENT_3D('',#62172,#26421,#26422);
#21841=AXIS2_PLACEMENT_3D('',#62175,#26423,#26424);
#21842=AXIS2_PLACEMENT_3D('',#62177,#26425,#26426);
#21843=AXIS2_PLACEMENT_3D('',#62178,#26427,#26428);
#21844=AXIS2_PLACEMENT_3D('',#62179,#26429,#26430);
#21845=AXIS2_PLACEMENT_3D('',#62182,#26431,#26432);
#21846=AXIS2_PLACEMENT_3D('',#62185,#26435,#26436);
#21847=AXIS2_PLACEMENT_3D('',#62187,#26437,#26438);
#21848=AXIS2_PLACEMENT_3D('',#62188,#26439,#26440);
#21849=AXIS2_PLACEMENT_3D('',#62189,#26441,#26442);
#21850=AXIS2_PLACEMENT_3D('',#62191,#26444,#26445);
#21851=AXIS2_PLACEMENT_3D('',#62194,#26448,#26449);
#21852=AXIS2_PLACEMENT_3D('',#62197,#26452,#26453);
#21853=AXIS2_PLACEMENT_3D('',#62198,#26454,#26455);
#21854=AXIS2_PLACEMENT_3D('',#62200,#26456,#26457);
#21855=AXIS2_PLACEMENT_3D('',#62202,#26458,#26459);
#21856=AXIS2_PLACEMENT_3D('',#62204,#26461,#26462);
#21857=AXIS2_PLACEMENT_3D('',#62207,#26463,#26464);
#21858=AXIS2_PLACEMENT_3D('',#62211,#26466,#26467);
#21859=AXIS2_PLACEMENT_3D('',#62213,#26469,#26470);
#21860=AXIS2_PLACEMENT_3D('',#62215,#26471,#26472);
#21861=AXIS2_PLACEMENT_3D('',#62216,#26473,#26474);
#21862=AXIS2_PLACEMENT_3D('',#62217,#26475,#26476);
#21863=AXIS2_PLACEMENT_3D('',#62219,#26477,#26478);
#21864=AXIS2_PLACEMENT_3D('',#62220,#26479,#26480);
#21865=AXIS2_PLACEMENT_3D('',#62221,#26481,#26482);
#21866=AXIS2_PLACEMENT_3D('',#62225,#26484,#26485);
#21867=AXIS2_PLACEMENT_3D('',#62227,#26487,#26488);
#21868=AXIS2_PLACEMENT_3D('',#62231,#26490,#26491);
#21869=AXIS2_PLACEMENT_3D('',#62233,#26493,#26494);
#21870=AXIS2_PLACEMENT_3D('',#62237,#26497,#26498);
#21871=AXIS2_PLACEMENT_3D('',#62257,#26500,#26501);
#21872=AXIS2_PLACEMENT_3D('',#62261,#26503,#26504);
#21873=AXIS2_PLACEMENT_3D('',#62263,#26506,#26507);
#21874=AXIS2_PLACEMENT_3D('',#62264,#26508,#26509);
#21875=AXIS2_PLACEMENT_3D('',#62268,#26511,#26512);
#21876=AXIS2_PLACEMENT_3D('',#62270,#26514,#26515);
#21877=AXIS2_PLACEMENT_3D('',#62273,#26516,#26517);
#21878=AXIS2_PLACEMENT_3D('',#62276,#26519,#26520);
#21879=AXIS2_PLACEMENT_3D('',#62296,#26523,#26524);
#21880=AXIS2_PLACEMENT_3D('',#62297,#26525,#26526);
#21881=AXIS2_PLACEMENT_3D('',#62298,#26527,#26528);
#21882=AXIS2_PLACEMENT_3D('',#62299,#26529,#26530);
#21883=AXIS2_PLACEMENT_3D('',#62302,#26532,#26533);
#21884=AXIS2_PLACEMENT_3D('',#62305,#26535,#26536);
#21885=AXIS2_PLACEMENT_3D('',#62306,#26537,#26538);
#21886=AXIS2_PLACEMENT_3D('',#62307,#26539,#26540);
#21887=AXIS2_PLACEMENT_3D('',#62309,#26542,#26543);
#21888=AXIS2_PLACEMENT_3D('',#62311,#26545,#26546);
#21889=AXIS2_PLACEMENT_3D('',#62315,#26549,#26550);
#21890=AXIS2_PLACEMENT_3D('',#62317,#26551,#26552);
#21891=AXIS2_PLACEMENT_3D('',#62320,#26554,#26555);
#21892=AXIS2_PLACEMENT_3D('',#62321,#26556,#26557);
#21893=AXIS2_PLACEMENT_3D('',#62330,#26558,#26559);
#21894=AXIS2_PLACEMENT_3D('',#62332,#26560,#26561);
#21895=AXIS2_PLACEMENT_3D('',#62333,#26562,#26563);
#21896=AXIS2_PLACEMENT_3D('',#62334,#26564,#26565);
#21897=AXIS2_PLACEMENT_3D('',#62335,#26566,#26567);
#21898=AXIS2_PLACEMENT_3D('',#62337,#26568,#26569);
#21899=AXIS2_PLACEMENT_3D('',#62361,#26570,#26571);
#21900=AXIS2_PLACEMENT_3D('',#62385,#26572,#26573);
#21901=AXIS2_PLACEMENT_3D('',#62392,#26574,#26575);
#21902=AXIS2_PLACEMENT_3D('',#62393,#26576,#26577);
#21903=AXIS2_PLACEMENT_3D('',#62397,#26579,#26580);
#21904=AXIS2_PLACEMENT_3D('',#62401,#26582,#26583);
#21905=AXIS2_PLACEMENT_3D('',#62409,#26590,#26591);
#21906=AXIS2_PLACEMENT_3D('',#62410,#26592,#26593);
#21907=AXIS2_PLACEMENT_3D('',#62414,#26595,#26596);
#21908=AXIS2_PLACEMENT_3D('',#62415,#26597,#26598);
#21909=AXIS2_PLACEMENT_3D('',#62416,#26599,#26600);
#21910=AXIS2_PLACEMENT_3D('',#62418,#26601,#26602);
#21911=AXIS2_PLACEMENT_3D('',#62420,#26603,#26604);
#21912=AXIS2_PLACEMENT_3D('',#62422,#26605,#26606);
#21913=AXIS2_PLACEMENT_3D('',#62423,#26607,#26608);
#21914=AXIS2_PLACEMENT_3D('',#62424,#26609,#26610);
#21915=AXIS2_PLACEMENT_3D('',#62428,#26612,#26613);
#21916=AXIS2_PLACEMENT_3D('',#62429,#26614,#26615);
#21917=AXIS2_PLACEMENT_3D('',#62430,#26616,#26617);
#21918=AXIS2_PLACEMENT_3D('',#62432,#26618,#26619);
#21919=AXIS2_PLACEMENT_3D('',#62433,#26620,#26621);
#21920=AXIS2_PLACEMENT_3D('',#62434,#26622,#26623);
#21921=AXIS2_PLACEMENT_3D('',#62435,#26624,#26625);
#21922=AXIS2_PLACEMENT_3D('',#62436,#26626,#26627);
#21923=AXIS2_PLACEMENT_3D('',#62437,#26628,#26629);
#21924=AXIS2_PLACEMENT_3D('',#62439,#26631,#26632);
#21925=AXIS2_PLACEMENT_3D('',#62440,#26633,#26634);
#21926=AXIS2_PLACEMENT_3D('',#62441,#26635,#26636);
#21927=AXIS2_PLACEMENT_3D('',#62442,#26637,#26638);
#21928=AXIS2_PLACEMENT_3D('',#62443,#26639,#26640);
#21929=AXIS2_PLACEMENT_3D('',#62445,#26641,#26642);
#21930=AXIS2_PLACEMENT_3D('',#62449,#26644,#26645);
#21931=AXIS2_PLACEMENT_3D('',#62451,#26647,#26648);
#21932=AXIS2_PLACEMENT_3D('',#62453,#26649,#26650);
#21933=AXIS2_PLACEMENT_3D('',#62457,#26652,#26653);
#21934=AXIS2_PLACEMENT_3D('',#62459,#26655,#26656);
#21935=AXIS2_PLACEMENT_3D('',#62461,#26657,#26658);
#21936=AXIS2_PLACEMENT_3D('',#62465,#26660,#26661);
#21937=AXIS2_PLACEMENT_3D('',#62467,#26663,#26664);
#21938=AXIS2_PLACEMENT_3D('',#62469,#26665,#26666);
#21939=AXIS2_PLACEMENT_3D('',#62470,#26667,#26668);
#21940=AXIS2_PLACEMENT_3D('',#62471,#26669,#26670);
#21941=AXIS2_PLACEMENT_3D('',#62472,#26671,#26672);
#21942=AXIS2_PLACEMENT_3D('',#62473,#26673,#26674);
#21943=AXIS2_PLACEMENT_3D('',#62474,#26675,#26676);
#21944=AXIS2_PLACEMENT_3D('',#62475,#26677,#26678);
#21945=AXIS2_PLACEMENT_3D('',#62479,#26681,#26682);
#21946=AXIS2_PLACEMENT_3D('',#62482,#26684,#26685);
#21947=AXIS2_PLACEMENT_3D('',#62483,#26686,#26687);
#21948=AXIS2_PLACEMENT_3D('',#62487,#26690,#26691);
#21949=AXIS2_PLACEMENT_3D('',#62490,#26693,#26694);
#21950=AXIS2_PLACEMENT_3D('',#62491,#26695,#26696);
#21951=AXIS2_PLACEMENT_3D('',#62495,#26699,#26700);
#21952=AXIS2_PLACEMENT_3D('',#62497,#26701,#26702);
#21953=AXIS2_PLACEMENT_3D('',#62499,#26703,#26704);
#21954=AXIS2_PLACEMENT_3D('',#62500,#26705,#26706);
#21955=AXIS2_PLACEMENT_3D('',#62501,#26707,#26708);
#21956=AXIS2_PLACEMENT_3D('',#62505,#26710,#26711);
#21957=AXIS2_PLACEMENT_3D('',#62506,#26712,#26713);
#21958=AXIS2_PLACEMENT_3D('',#62507,#26714,#26715);
#21959=AXIS2_PLACEMENT_3D('',#62509,#26716,#26717);
#21960=AXIS2_PLACEMENT_3D('',#62511,#26718,#26719);
#21961=AXIS2_PLACEMENT_3D('',#62512,#26720,#26721);
#21962=AXIS2_PLACEMENT_3D('',#62513,#26722,#26723);
#21963=AXIS2_PLACEMENT_3D('',#62515,#26725,#26726);
#21964=AXIS2_PLACEMENT_3D('',#62517,#26727,#26728);
#21965=AXIS2_PLACEMENT_3D('',#62518,#26729,#26730);
#21966=AXIS2_PLACEMENT_3D('',#62519,#26731,#26732);
#21967=AXIS2_PLACEMENT_3D('',#62521,#26733,#26734);
#21968=AXIS2_PLACEMENT_3D('',#62522,#26735,#26736);
#21969=AXIS2_PLACEMENT_3D('',#62523,#26737,#26738);
#21970=AXIS2_PLACEMENT_3D('',#62525,#26739,#26740);
#21971=AXIS2_PLACEMENT_3D('',#62526,#26741,#26742);
#21972=AXIS2_PLACEMENT_3D('',#62528,#26743,#26744);
#21973=AXIS2_PLACEMENT_3D('',#62531,#26746,#26747);
#21974=AXIS2_PLACEMENT_3D('',#62532,#26748,#26749);
#21975=AXIS2_PLACEMENT_3D('',#62533,#26750,#26751);
#21976=AXIS2_PLACEMENT_3D('',#62534,#26752,#26753);
#21977=AXIS2_PLACEMENT_3D('',#62538,#26755,#26756);
#21978=AXIS2_PLACEMENT_3D('',#62540,#26758,#26759);
#21979=AXIS2_PLACEMENT_3D('',#62544,#26762,#26763);
#21980=AXIS2_PLACEMENT_3D('',#62545,#26764,#26765);
#21981=AXIS2_PLACEMENT_3D('',#62546,#26766,#26767);
#21982=AXIS2_PLACEMENT_3D('',#62548,#26769,#26770);
#21983=AXIS2_PLACEMENT_3D('',#62549,#26771,#26772);
#21984=AXIS2_PLACEMENT_3D('',#62550,#26773,#26774);
#21985=AXIS2_PLACEMENT_3D('',#62552,#26776,#26777);
#21986=AXIS2_PLACEMENT_3D('',#62553,#26778,#26779);
#21987=AXIS2_PLACEMENT_3D('',#62554,#26780,#26781);
#21988=AXIS2_PLACEMENT_3D('',#62555,#26782,#26783);
#21989=AXIS2_PLACEMENT_3D('',#62556,#26784,#26785);
#21990=AXIS2_PLACEMENT_3D('',#62558,#26787,#26788);
#21991=AXIS2_PLACEMENT_3D('',#62560,#26789,#26790);
#21992=AXIS2_PLACEMENT_3D('',#62562,#26791,#26792);
#21993=AXIS2_PLACEMENT_3D('',#62563,#26793,#26794);
#21994=AXIS2_PLACEMENT_3D('',#62564,#26795,#26796);
#21995=AXIS2_PLACEMENT_3D('',#62567,#26797,#26798);
#21996=AXIS2_PLACEMENT_3D('',#62569,#26800,#26801);
#21997=AXIS2_PLACEMENT_3D('',#62570,#26802,#26803);
#21998=AXIS2_PLACEMENT_3D('',#62572,#26804,#26805);
#21999=AXIS2_PLACEMENT_3D('',#62573,#26806,#26807);
#22000=AXIS2_PLACEMENT_3D('',#62574,#26808,#26809);
#22001=AXIS2_PLACEMENT_3D('',#62576,#26810,#26811);
#22002=AXIS2_PLACEMENT_3D('',#62577,#26812,#26813);
#22003=AXIS2_PLACEMENT_3D('',#62579,#26815,#26816);
#22004=AXIS2_PLACEMENT_3D('',#62580,#26817,#26818);
#22005=AXIS2_PLACEMENT_3D('',#62581,#26819,#26820);
#22006=AXIS2_PLACEMENT_3D('',#62582,#26821,#26822);
#22007=AXIS2_PLACEMENT_3D('',#62583,#26823,#26824);
#22008=AXIS2_PLACEMENT_3D('',#62584,#26825,#26826);
#26259=DIRECTION('axis',(0.,0.,1.));
#26260=DIRECTION('refdir',(1.,0.,0.));
#26261=DIRECTION('center_axis',(0.,-1.,1.63268091856641E-16));
#26262=DIRECTION('ref_axis',(-0.707106781186548,0.,0.707106781186548));
#26263=DIRECTION('',(0.,-1.,1.63268091856641E-16));
#26264=DIRECTION('center_axis',(0.,1.,0.));
#26265=DIRECTION('ref_axis',(-1.,0.,0.));
#26266=DIRECTION('',(0.,1.,-1.63268091856641E-16));
#26267=DIRECTION('center_axis',(-0.707106781186548,-0.707106781186548,0.));
#26268=DIRECTION('ref_axis',(-0.707106781186548,0.707106781186548,-1.2266347333467E-16));
#26269=DIRECTION('',(0.,1.,-1.63268091856641E-16));
#26270=DIRECTION('center_axis',(0.,0.,-1.));
#26271=DIRECTION('ref_axis',(-0.707106781186548,-0.707106781186548,0.));
#26272=DIRECTION('',(0.,0.,1.));
#26273=DIRECTION('center_axis',(0.,0.,-1.));
#26274=DIRECTION('ref_axis',(0.,-1.,0.));
#26275=DIRECTION('',(0.,0.,-1.));
#26276=DIRECTION('center_axis',(-0.707106781186548,0.,0.707106781186548));
#26277=DIRECTION('ref_axis',(0.707106781186547,0.,0.707106781186547));
#26278=DIRECTION('center_axis',(-0.408248290463863,-0.816496580927726,0.408248290463863));
#26279=DIRECTION('ref_axis',(0.577350269189627,-0.577350269189623,-0.577350269189628));
#26280=DIRECTION('center_axis',(0.,0.,-1.));
#26281=DIRECTION('ref_axis',(0.,-1.,0.));
#26282=DIRECTION('center_axis',(1.,0.,0.));
#26283=DIRECTION('ref_axis',(0.,0.,-1.));
#26284=DIRECTION('center_axis',(0.,-1.,0.));
#26285=DIRECTION('ref_axis',(1.,0.,0.));
#26286=DIRECTION('center_axis',(1.,0.,0.));
#26287=DIRECTION('ref_axis',(0.,-0.707106781186548,-0.707106781186548));
#26288=DIRECTION('',(1.,0.,0.));
#26289=DIRECTION('',(-1.,0.,0.));
#26290=DIRECTION('center_axis',(0.,1.,-1.63268091856641E-16));
#26291=DIRECTION('ref_axis',(0.707106781186548,0.,-0.707106781186548));
#26292=DIRECTION('center_axis',(0.,-1.,0.));
#26293=DIRECTION('ref_axis',(0.,0.,-1.));
#26294=DIRECTION('',(0.,-1.,1.63268091856641E-16));
#26295=DIRECTION('',(0.,1.,-1.63268091856641E-16));
#26296=DIRECTION('center_axis',(0.408248290463861,-0.816496580927727,-0.408248290463863));
#26297=DIRECTION('ref_axis',(0.577350269189626,0.577350269189624,-0.577350269189628));
#26298=DIRECTION('center_axis',(1.,0.,0.));
#26299=DIRECTION('ref_axis',(0.,0.707106781186546,-0.707106781186549));
#26300=DIRECTION('center_axis',(0.,0.,-1.));
#26301=DIRECTION('ref_axis',(0.707106781186549,0.707106781186546,0.));
#26302=DIRECTION('center_axis',(-0.408248290463861,-0.816496580927727,-0.408248290463863));
#26303=DIRECTION('ref_axis',(0.577350269189626,-0.577350269189624,0.577350269189628));
#26304=DIRECTION('center_axis',(-1.38777878078145E-15,0.,1.));
#26305=DIRECTION('ref_axis',(0.,-1.,0.));
#26306=DIRECTION('center_axis',(0.,-1.,1.63268091856641E-16));
#26307=DIRECTION('ref_axis',(0.707106781186548,0.,0.707106781186548));
#26308=DIRECTION('center_axis',(1.,0.,0.));
#26309=DIRECTION('ref_axis',(0.,-0.707106781186549,0.707106781186546));
#26310=DIRECTION('center_axis',(0.,0.,-1.));
#26311=DIRECTION('ref_axis',(0.707106781186548,-0.707106781186548,0.));
#26312=DIRECTION('',(0.,0.,-1.));
#26313=DIRECTION('',(0.,0.,1.));
#26314=DIRECTION('center_axis',(0.408248290463861,-0.816496580927727,-0.408248290463862));
#26315=DIRECTION('ref_axis',(-0.577350269189626,-0.577350269189624,0.577350269189627));
#26316=DIRECTION('center_axis',(-1.,0.,0.));
#26317=DIRECTION('ref_axis',(0.,-0.707106781186549,0.707106781186546));
#26318=DIRECTION('center_axis',(1.,0.,0.));
#26319=DIRECTION('ref_axis',(0.,0.707106781186548,0.707106781186548));
#26320=DIRECTION('',(1.,0.,0.));
#26321=DIRECTION('center_axis',(1.,0.,0.));
#26322=DIRECTION('ref_axis',(0.,0.,1.));
#26323=DIRECTION('',(-1.,0.,0.));
#26324=DIRECTION('center_axis',(-1.,0.,0.));
#26325=DIRECTION('ref_axis',(0.,0.707106781186548,0.707106781186548));
#26326=DIRECTION('center_axis',(0.,1.63268091856641E-16,1.));
#26327=DIRECTION('ref_axis',(0.,-1.,1.63268091856641E-16));
#26328=DIRECTION('',(-1.,0.,0.));
#26329=DIRECTION('',(0.,-1.,1.63268091856641E-16));
#26330=DIRECTION('center_axis',(0.,-1.,0.));
#26331=DIRECTION('ref_axis',(0.,0.,-1.));
#26332=DIRECTION('',(1.,0.,0.));
#26333=DIRECTION('center_axis',(1.,0.,0.));
#26334=DIRECTION('ref_axis',(0.,-0.707106781186548,0.707106781186548));
#26335=DIRECTION('center_axis',(1.,0.,0.));
#26336=DIRECTION('ref_axis',(0.,0.707106781186548,-0.707106781186548));
#26337=DIRECTION('',(-1.,0.,0.));
#26338=DIRECTION('center_axis',(-1.,0.,0.));
#26339=DIRECTION('ref_axis',(0.,0.707106781186548,-0.707106781186548));
#26340=DIRECTION('',(1.,0.,0.));
#26341=DIRECTION('center_axis',(-0.816496580927727,0.40824829046386,0.408248290463864));
#26342=DIRECTION('ref_axis',(0.577350269189627,0.577350269189624,0.577350269189627));
#26343=DIRECTION('center_axis',(0.,0.,1.));
#26344=DIRECTION('ref_axis',(0.,1.,0.));
#26345=DIRECTION('center_axis',(0.,1.,0.));
#26346=DIRECTION('ref_axis',(1.,0.,0.));
#26347=DIRECTION('center_axis',(0.,-1.,1.63268091856641E-16));
#26348=DIRECTION('ref_axis',(0.707106781186548,0.,0.707106781186548));
#26349=DIRECTION('',(0.,1.,-1.63268091856641E-16));
#26350=DIRECTION('center_axis',(0.,0.,1.));
#26351=DIRECTION('ref_axis',(0.707106781186548,0.707106781186548,0.));
#26352=DIRECTION('',(0.,0.,1.));
#26353=DIRECTION('',(0.,0.,-1.));
#26354=DIRECTION('center_axis',(1.,0.,0.));
#26355=DIRECTION('ref_axis',(0.,0.,-1.));
#26356=DIRECTION('center_axis',(1.,0.,0.));
#26357=DIRECTION('ref_axis',(0.,0.,-1.));
#26358=DIRECTION('center_axis',(1.,0.,0.));
#26359=DIRECTION('ref_axis',(0.,0.,-1.));
#26360=DIRECTION('',(0.,1.,-1.63268091856641E-16));
#26361=DIRECTION('center_axis',(0.,0.,1.));
#26362=DIRECTION('ref_axis',(-0.707106781186548,0.707106781186548,0.));
#26363=DIRECTION('',(0.,0.,1.));
#26364=DIRECTION('center_axis',(0.,0.,-1.));
#26365=DIRECTION('ref_axis',(-1.,0.,0.));
#26366=DIRECTION('',(0.,0.,-1.));
#26367=DIRECTION('center_axis',(-0.707106781186548,0.,0.707106781186548));
#26368=DIRECTION('ref_axis',(-0.707106781186547,0.,-0.707106781186547));
#26369=DIRECTION('',(0.,0.,-1.));
#26370=DIRECTION('center_axis',(0.,-1.,0.));
#26371=DIRECTION('ref_axis',(0.707106781186548,0.,0.707106781186548));
#26372=DIRECTION('center_axis',(0.,1.,0.));
#26373=DIRECTION('ref_axis',(0.,0.,1.));
#26374=DIRECTION('',(0.,1.,0.));
#26375=DIRECTION('center_axis',(0.,-1.,0.));
#26376=DIRECTION('ref_axis',(1.,0.,0.));
#26377=DIRECTION('',(0.,-1.,0.));
#26378=DIRECTION('center_axis',(0.408248290463864,-0.816496580927727,0.40824829046386));
#26379=DIRECTION('ref_axis',(0.577350269189626,0.577350269189627,0.577350269189624));
#26380=DIRECTION('center_axis',(0.,0.,1.));
#26381=DIRECTION('ref_axis',(0.707106781186548,0.707106781186548,0.));
#26382=DIRECTION('center_axis',(1.,0.,0.));
#26383=DIRECTION('ref_axis',(0.,0.707106781186546,0.707106781186549));
#26384=DIRECTION('center_axis',(0.,-1.,0.));
#26385=DIRECTION('ref_axis',(-0.707106781186548,0.,0.707106781186548));
#26386=DIRECTION('',(0.,1.,0.));
#26387=DIRECTION('center_axis',(0.,-1.,0.));
#26388=DIRECTION('ref_axis',(0.,0.,1.));
#26389=DIRECTION('',(0.,-1.,0.));
#26390=DIRECTION('center_axis',(-0.707106781186547,0.707106781186548,0.));
#26391=DIRECTION('ref_axis',(0.707106781186548,0.707106781186547,0.));
#26392=DIRECTION('center_axis',(1.,0.,0.));
#26393=DIRECTION('ref_axis',(0.,-0.707106781186548,0.707106781186548));
#26394=DIRECTION('',(1.,0.,0.));
#26395=DIRECTION('center_axis',(-1.,0.,0.));
#26396=DIRECTION('ref_axis',(0.,-1.,0.));
#26397=DIRECTION('',(-1.,0.,0.));
#26398=DIRECTION('center_axis',(-0.408248290463863,-0.816496580927727,-0.40824829046386));
#26399=DIRECTION('ref_axis',(0.577350269189627,-0.577350269189627,0.577350269189624));
#26400=DIRECTION('center_axis',(0.,0.,1.));
#26401=DIRECTION('ref_axis',(0.707106781186548,-0.707106781186548,0.));
#26402=DIRECTION('center_axis',(-0.408248290463865,-0.816496580927727,0.40824829046386));
#26403=DIRECTION('ref_axis',(-0.577350269189626,0.577350269189627,0.577350269189624));
#26404=DIRECTION('center_axis',(-1.,0.,0.));
#26405=DIRECTION('ref_axis',(0.,0.707106781186546,0.707106781186549));
#26406=DIRECTION('center_axis',(1.,0.,0.));
#26407=DIRECTION('ref_axis',(0.,0.707106781186548,-0.707106781186548));
#26408=DIRECTION('',(1.,0.,0.));
#26409=DIRECTION('center_axis',(1.,0.,0.));
#26410=DIRECTION('ref_axis',(0.,1.,0.));
#26411=DIRECTION('',(-1.,0.,0.));
#26412=DIRECTION('center_axis',(-1.,0.,0.));
#26413=DIRECTION('ref_axis',(0.,0.707106781186548,-0.707106781186548));
#26414=DIRECTION('center_axis',(0.,1.,0.));
#26415=DIRECTION('ref_axis',(0.,0.,1.));
#26416=DIRECTION('',(-1.,0.,0.));
#26417=DIRECTION('',(0.,0.,1.));
#26418=DIRECTION('center_axis',(1.,0.,0.));
#26419=DIRECTION('ref_axis',(0.,0.707106781186548,0.707106781186548));
#26420=DIRECTION('',(1.,0.,0.));
#26421=DIRECTION('center_axis',(-0.408248290463864,-0.816496580927727,0.40824829046386));
#26422=DIRECTION('ref_axis',(0.577350269189627,-0.577350269189627,-0.577350269189624));
#26423=DIRECTION('center_axis',(0.,0.,-1.));
#26424=DIRECTION('ref_axis',(0.,-1.,0.));
#26425=DIRECTION('center_axis',(1.,0.,0.));
#26426=DIRECTION('ref_axis',(0.,0.,-1.));
#26427=DIRECTION('center_axis',(0.,-1.,0.));
#26428=DIRECTION('ref_axis',(1.,0.,0.));
#26429=DIRECTION('center_axis',(1.,0.,0.));
#26430=DIRECTION('ref_axis',(0.,-0.707106781186548,-0.707106781186548));
#26431=DIRECTION('center_axis',(-1.,0.,0.));
#26432=DIRECTION('ref_axis',(0.,-0.707106781186548,-0.707106781186548));
#26433=DIRECTION('',(1.,0.,0.));
#26434=DIRECTION('',(-1.,0.,0.));
#26435=DIRECTION('center_axis',(0.408248290463863,-0.816496580927727,-0.40824829046386));
#26436=DIRECTION('ref_axis',(0.577350269189627,0.577350269189628,-0.577350269189623));
#26437=DIRECTION('center_axis',(0.,1.,0.));
#26438=DIRECTION('ref_axis',(0.,0.,-1.));
#26439=DIRECTION('center_axis',(0.,0.,-1.));
#26440=DIRECTION('ref_axis',(1.,0.,0.));
#26441=DIRECTION('center_axis',(0.,0.,1.));
#26442=DIRECTION('ref_axis',(0.707106781186548,0.707106781186548,0.));
#26443=DIRECTION('',(0.,0.,-1.));
#26444=DIRECTION('center_axis',(0.,1.,0.));
#26445=DIRECTION('ref_axis',(0.707106781186548,0.,-0.707106781186548));
#26446=DIRECTION('',(0.,-1.,0.));
#26447=DIRECTION('',(0.,1.,0.));
#26448=DIRECTION('center_axis',(0.,0.,-1.));
#26449=DIRECTION('ref_axis',(0.707106781186548,-0.707106781186548,0.));
#26450=DIRECTION('',(0.,0.,-1.));
#26451=DIRECTION('',(0.,0.,1.));
#26452=DIRECTION('center_axis',(1.,0.,0.));
#26453=DIRECTION('ref_axis',(0.,0.,-1.));
#26454=DIRECTION('center_axis',(1.,0.,0.));
#26455=DIRECTION('ref_axis',(0.,0.,-1.));
#26456=DIRECTION('center_axis',(1.,0.,0.));
#26457=DIRECTION('ref_axis',(0.,0.,-1.));
#26458=DIRECTION('center_axis',(1.,0.,0.));
#26459=DIRECTION('ref_axis',(0.,0.,-1.));
#26460=DIRECTION('',(0.,0.,-1.));
#26461=DIRECTION('center_axis',(0.,0.,1.));
#26462=DIRECTION('ref_axis',(0.707106781186548,0.707106781186548,0.));
#26463=DIRECTION('center_axis',(0.,0.,1.));
#26464=DIRECTION('ref_axis',(1.,0.,0.));
#26465=DIRECTION('',(0.,0.,1.));
#26466=DIRECTION('center_axis',(0.,0.,-1.));
#26467=DIRECTION('ref_axis',(0.,1.,0.));
#26468=DIRECTION('',(0.,0.,-1.));
#26469=DIRECTION('center_axis',(-0.816496580927727,0.40824829046386,0.408248290463864));
#26470=DIRECTION('ref_axis',(0.577350269189627,0.577350269189624,0.577350269189627));
#26471=DIRECTION('center_axis',(1.,0.,0.));
#26472=DIRECTION('ref_axis',(0.,0.707106781186549,0.707106781186546));
#26473=DIRECTION('center_axis',(0.,1.,0.));
#26474=DIRECTION('ref_axis',(0.707106781186548,0.,0.707106781186548));
#26475=DIRECTION('center_axis',(-0.816496580927727,0.40824829046386,-0.408248290463864));
#26476=DIRECTION('ref_axis',(0.577350269189627,0.577350269189624,-0.577350269189627));
#26477=DIRECTION('center_axis',(0.,1.,0.));
#26478=DIRECTION('ref_axis',(0.707106781186548,0.,-0.707106781186548));
#26479=DIRECTION('center_axis',(1.,0.,0.));
#26480=DIRECTION('ref_axis',(0.,0.707106781186549,-0.707106781186546));
#26481=DIRECTION('center_axis',(1.,0.,0.));
#26482=DIRECTION('ref_axis',(0.,0.707106781186548,-0.707106781186548));
#26483=DIRECTION('',(-1.,0.,0.));
#26484=DIRECTION('center_axis',(-1.,0.,0.));
#26485=DIRECTION('ref_axis',(0.,0.707106781186549,-0.707106781186546));
#26486=DIRECTION('',(1.,0.,0.));
#26487=DIRECTION('center_axis',(0.,1.,0.));
#26488=DIRECTION('ref_axis',(0.707106781186548,0.,-0.707106781186548));
#26489=DIRECTION('',(0.,-1.,0.));
#26490=DIRECTION('center_axis',(0.,1.,0.));
#26491=DIRECTION('ref_axis',(1.,0.,0.));
#26492=DIRECTION('',(0.,1.,0.));
#26493=DIRECTION('center_axis',(1.,0.,0.));
#26494=DIRECTION('ref_axis',(0.,0.,-1.));
#26495=DIRECTION('',(0.,1.,0.));
#26496=DIRECTION('',(0.,0.,1.));
#26497=DIRECTION('center_axis',(0.,1.,0.));
#26498=DIRECTION('ref_axis',(-0.707106781186548,0.,-0.707106781186548));
#26499=DIRECTION('',(0.,1.,0.));
#26500=DIRECTION('center_axis',(0.,-1.,0.));
#26501=DIRECTION('ref_axis',(-1.,0.,0.));
#26502=DIRECTION('',(0.,-1.,0.));
#26503=DIRECTION('center_axis',(-0.707106781186548,0.707106781186548,0.));
#26504=DIRECTION('ref_axis',(-0.707106781186547,-0.707106781186547,0.));
#26505=DIRECTION('',(0.,-1.,0.));
#26506=DIRECTION('center_axis',(0.,0.,1.));
#26507=DIRECTION('ref_axis',(-0.707106781186548,0.707106781186548,0.));
#26508=DIRECTION('center_axis',(0.,0.,1.));
#26509=DIRECTION('ref_axis',(0.,1.,0.));
#26510=DIRECTION('',(0.,0.,1.));
#26511=DIRECTION('center_axis',(0.,0.,-1.));
#26512=DIRECTION('ref_axis',(-1.,0.,0.));
#26513=DIRECTION('',(0.,0.,-1.));
#26514=DIRECTION('center_axis',(0.,-1.,0.));
#26515=DIRECTION('ref_axis',(-0.707106781186548,0.,0.707106781186548));
#26516=DIRECTION('center_axis',(-0.707106781186548,0.707106781186548,0.));
#26517=DIRECTION('ref_axis',(-0.707106781186547,-0.707106781186547,0.));
#26518=DIRECTION('',(0.,1.,0.));
#26519=DIRECTION('center_axis',(0.,-1.,0.));
#26520=DIRECTION('ref_axis',(0.,0.,1.));
#26521=DIRECTION('',(0.,-1.,0.));
#26522=DIRECTION('',(0.,1.,0.));
#26523=DIRECTION('center_axis',(-0.816496580927727,-0.40824829046386,-0.408248290463864));
#26524=DIRECTION('ref_axis',(-0.577350269189628,0.577350269189623,0.577350269189627));
#26525=DIRECTION('center_axis',(-1.,0.,0.));
#26526=DIRECTION('ref_axis',(0.,0.707106781186549,0.707106781186546));
#26527=DIRECTION('center_axis',(-0.816496580927727,-0.40824829046386,0.408248290463864));
#26528=DIRECTION('ref_axis',(-0.577350269189628,0.577350269189623,-0.577350269189627));
#26529=DIRECTION('center_axis',(1.,0.,0.));
#26530=DIRECTION('ref_axis',(0.,-0.707106781186548,-0.707106781186548));
#26531=DIRECTION('',(1.,0.,0.));
#26532=DIRECTION('center_axis',(1.,0.,0.));
#26533=DIRECTION('ref_axis',(0.,-0.707106781186546,-0.707106781186549));
#26534=DIRECTION('',(-1.,0.,0.));
#26535=DIRECTION('center_axis',(-1.,0.,0.));
#26536=DIRECTION('ref_axis',(0.,-0.707106781186548,-0.707106781186548));
#26537=DIRECTION('center_axis',(0.,0.,-1.));
#26538=DIRECTION('ref_axis',(0.,1.,0.));
#26539=DIRECTION('center_axis',(0.,1.,0.));
#26540=DIRECTION('ref_axis',(0.,0.,1.));
#26541=DIRECTION('',(-1.,0.,0.));
#26542=DIRECTION('center_axis',(1.,0.,0.));
#26543=DIRECTION('ref_axis',(0.,0.707106781186548,0.707106781186548));
#26544=DIRECTION('',(1.,0.,0.));
#26545=DIRECTION('center_axis',(0.,0.,1.));
#26546=DIRECTION('ref_axis',(0.,-1.,0.));
#26547=DIRECTION('',(-1.,0.,0.));
#26548=DIRECTION('',(0.,-1.,0.));
#26549=DIRECTION('center_axis',(1.,0.,0.));
#26550=DIRECTION('ref_axis',(0.,-0.707106781186548,0.707106781186548));
#26551=DIRECTION('center_axis',(-1.,0.,0.));
#26552=DIRECTION('ref_axis',(0.,-0.707106781186548,0.707106781186548));
#26553=DIRECTION('',(1.,0.,0.));
#26554=DIRECTION('center_axis',(1.,0.,0.));
#26555=DIRECTION('ref_axis',(0.,-1.,0.));
#26556=DIRECTION('center_axis',(1.,0.,0.));
#26557=DIRECTION('ref_axis',(0.,0.,-1.));
#26558=DIRECTION('center_axis',(0.,-1.,-1.22464679914735E-16));
#26559=DIRECTION('ref_axis',(0.,-1.22464679914735E-16,1.));
#26560=DIRECTION('center_axis',(1.,-3.67724725538251E-17,-3.65371805748965E-17));
#26561=DIRECTION('ref_axis',(0.,0.704833646806666,-0.709372631505625));
#26562=DIRECTION('center_axis',(1.,-3.67724725538251E-17,-3.65371805748965E-17));
#26563=DIRECTION('ref_axis',(0.,0.704833646806666,-0.709372631505625));
#26564=DIRECTION('center_axis',(1.,0.,0.));
#26565=DIRECTION('ref_axis',(0.,0.,-1.));
#26566=DIRECTION('center_axis',(1.,0.,0.));
#26567=DIRECTION('ref_axis',(0.,0.,-1.));
#26568=DIRECTION('center_axis',(1.,0.,0.));
#26569=DIRECTION('ref_axis',(0.,0.,-1.));
#26570=DIRECTION('center_axis',(1.,0.,0.));
#26571=DIRECTION('ref_axis',(0.,0.,-1.));
#26572=DIRECTION('center_axis',(-1.,0.,0.));
#26573=DIRECTION('ref_axis',(0.,0.704833646806666,-0.709372631505625));
#26574=DIRECTION('center_axis',(1.,0.,0.));
#26575=DIRECTION('ref_axis',(0.,0.,-1.));
#26576=DIRECTION('center_axis',(1.,0.,0.));
#26577=DIRECTION('ref_axis',(0.,0.,-1.));
#26578=DIRECTION('',(0.,0.,1.));
#26579=DIRECTION('center_axis',(-1.,0.,0.));
#26580=DIRECTION('ref_axis',(0.,-0.707106781186548,0.707106781186548));
#26581=DIRECTION('',(0.,1.,0.));
#26582=DIRECTION('center_axis',(-1.,0.,0.));
#26583=DIRECTION('ref_axis',(0.,0.707106781186548,0.707106781186548));
#26584=DIRECTION('',(0.,-1.63268091856641E-16,-1.));
#26585=DIRECTION('',(0.,0.,1.));
#26586=DIRECTION('',(0.,-1.,0.));
#26587=DIRECTION('',(0.,0.,1.));
#26588=DIRECTION('',(0.,0.,-1.));
#26589=DIRECTION('',(0.,-1.,1.63268091856641E-16));
#26590=DIRECTION('center_axis',(1.,0.,0.));
#26591=DIRECTION('ref_axis',(0.,1.,-1.82855839818329E-16));
#26592=DIRECTION('center_axis',(-1.,0.,0.));
#26593=DIRECTION('ref_axis',(0.,1.,0.));
#26594=DIRECTION('',(-0.707106781186546,-0.707106781186549,-8.65956056235495E-17));
#26595=DIRECTION('center_axis',(-1.,0.,0.));
#26596=DIRECTION('ref_axis',(0.,-1.,3.06161699786838E-17));
#26597=DIRECTION('center_axis',(-1.,0.,0.));
#26598=DIRECTION('ref_axis',(0.,-1.,3.06161699786838E-17));
#26599=DIRECTION('center_axis',(1.,0.,0.));
#26600=DIRECTION('ref_axis',(0.,0.,-1.));
#26601=DIRECTION('center_axis',(-1.,0.,0.));
#26602=DIRECTION('ref_axis',(0.,-1.,1.83697019872103E-16));
#26603=DIRECTION('center_axis',(0.,-1.,-1.22464679914735E-16));
#26604=DIRECTION('ref_axis',(0.,-1.22464679914735E-16,1.));
#26605=DIRECTION('center_axis',(1.,0.,0.));
#26606=DIRECTION('ref_axis',(0.,-1.,1.83697019872103E-16));
#26607=DIRECTION('center_axis',(1.,0.,0.));
#26608=DIRECTION('ref_axis',(0.,-1.,1.83697019872103E-16));
#26609=DIRECTION('center_axis',(1.,0.,0.));
#26610=DIRECTION('ref_axis',(0.,1.,0.));
#26611=DIRECTION('',(-1.,0.,0.));
#26612=DIRECTION('center_axis',(-1.,0.,0.));
#26613=DIRECTION('ref_axis',(0.,-1.,1.83697019872103E-16));
#26614=DIRECTION('center_axis',(-1.,0.,0.));
#26615=DIRECTION('ref_axis',(0.,-1.,1.83697019872103E-16));
#26616=DIRECTION('center_axis',(1.,0.,0.));
#26617=DIRECTION('ref_axis',(0.,0.,-1.));
#26618=DIRECTION('center_axis',(1.,0.,0.));
#26619=DIRECTION('ref_axis',(0.,0.,-1.));
#26620=DIRECTION('center_axis',(-0.816496580927728,-0.40824829046386,0.408248290463863));
#26621=DIRECTION('ref_axis',(0.577350269189627,-0.577350269189624,0.577350269189627));
#26622=DIRECTION('center_axis',(0.,-1.,0.));
#26623=DIRECTION('ref_axis',(0.,0.,1.));
#26624=DIRECTION('center_axis',(0.,0.,1.));
#26625=DIRECTION('ref_axis',(1.,0.,0.));
#26626=DIRECTION('center_axis',(0.,0.,-1.));
#26627=DIRECTION('ref_axis',(0.707106781186548,-0.707106781186548,0.));
#26628=DIRECTION('center_axis',(0.,0.,1.));
#26629=DIRECTION('ref_axis',(0.,-1.,0.));
#26630=DIRECTION('',(0.,0.,-1.));
#26631=DIRECTION('center_axis',(0.,-1.,0.));
#26632=DIRECTION('ref_axis',(0.707106781186548,0.,0.707106781186548));
#26633=DIRECTION('center_axis',(-0.816496580927727,-0.40824829046386,-0.408248290463864));
#26634=DIRECTION('ref_axis',(0.577350269189627,-0.577350269189624,-0.577350269189627));
#26635=DIRECTION('center_axis',(1.,0.,0.));
#26636=DIRECTION('ref_axis',(0.,0.,-1.));
#26637=DIRECTION('center_axis',(0.,-1.,0.));
#26638=DIRECTION('ref_axis',(0.,0.,-1.));
#26639=DIRECTION('center_axis',(0.,1.63268091856641E-16,1.));
#26640=DIRECTION('ref_axis',(-0.707106781186548,0.707106781186548,0.));
#26641=DIRECTION('center_axis',(-0.707106781186548,0.,-0.707106781186548));
#26642=DIRECTION('ref_axis',(-0.707106781186547,6.13317366673349E-17,0.707106781186547));
#26643=DIRECTION('',(0.,-1.63268091856641E-16,-1.));
#26644=DIRECTION('center_axis',(0.,0.,1.));
#26645=DIRECTION('ref_axis',(0.,1.,0.));
#26646=DIRECTION('',(0.,1.63268091856641E-16,1.));
#26647=DIRECTION('center_axis',(1.,0.,0.));
#26648=DIRECTION('ref_axis',(0.,0.707106781186548,-0.707106781186548));
#26649=DIRECTION('center_axis',(1.,0.,0.));
#26650=DIRECTION('ref_axis',(0.,0.,-1.));
#26651=DIRECTION('',(1.,0.,0.));
#26652=DIRECTION('center_axis',(-1.,0.,0.));
#26653=DIRECTION('ref_axis',(0.,1.,0.));
#26654=DIRECTION('',(-1.,0.,0.));
#26655=DIRECTION('center_axis',(0.,1.63268091856641E-16,1.));
#26656=DIRECTION('ref_axis',(0.707106781186548,0.707106781186548,0.));
#26657=DIRECTION('center_axis',(0.,0.,1.));
#26658=DIRECTION('ref_axis',(1.,0.,0.));
#26659=DIRECTION('',(0.,1.63268091856641E-16,1.));
#26660=DIRECTION('center_axis',(0.,0.,-1.));
#26661=DIRECTION('ref_axis',(0.,1.,0.));
#26662=DIRECTION('',(0.,-1.63268091856641E-16,-1.));
#26663=DIRECTION('center_axis',(-0.816496580927728,0.408248290463863,0.40824829046386));
#26664=DIRECTION('ref_axis',(0.577350269189626,0.577350269189628,0.577350269189624));
#26665=DIRECTION('center_axis',(1.,0.,0.));
#26666=DIRECTION('ref_axis',(0.,0.707106781186549,0.707106781186546));
#26667=DIRECTION('center_axis',(0.,1.,0.));
#26668=DIRECTION('ref_axis',(0.707106781186549,0.,0.707106781186546));
#26669=DIRECTION('center_axis',(0.408248290463864,-0.816496580927727,-0.40824829046386));
#26670=DIRECTION('ref_axis',(0.577350269189626,0.577350269189627,-0.577350269189624));
#26671=DIRECTION('center_axis',(0.,1.,0.));
#26672=DIRECTION('ref_axis',(0.707106781186546,0.,-0.707106781186549));
#26673=DIRECTION('center_axis',(-0.408248290463865,-0.816496580927727,-0.40824829046386));
#26674=DIRECTION('ref_axis',(-0.577350269189626,0.577350269189627,-0.577350269189624));
#26675=DIRECTION('center_axis',(0.,1.,0.));
#26676=DIRECTION('ref_axis',(-0.707106781186546,0.,-0.707106781186549));
#26677=DIRECTION('center_axis',(1.,0.,0.));
#26678=DIRECTION('ref_axis',(0.,0.,-1.));
#26679=DIRECTION('',(0.,1.,0.));
#26680=DIRECTION('',(0.,0.,-1.));
#26681=DIRECTION('center_axis',(0.,1.,0.));
#26682=DIRECTION('ref_axis',(-0.707106781186548,0.,-0.707106781186548));
#26683=DIRECTION('',(0.,-1.,0.));
#26684=DIRECTION('center_axis',(0.,1.,0.));
#26685=DIRECTION('ref_axis',(0.,0.,-1.));
#26686=DIRECTION('center_axis',(0.,0.,-1.));
#26687=DIRECTION('ref_axis',(0.,1.,0.));
#26688=DIRECTION('',(0.,1.,0.));
#26689=DIRECTION('',(1.,0.,0.));
#26690=DIRECTION('center_axis',(0.,1.,0.));
#26691=DIRECTION('ref_axis',(0.707106781186548,0.,-0.707106781186548));
#26692=DIRECTION('',(0.,-1.,0.));
#26693=DIRECTION('center_axis',(0.,-1.,0.));
#26694=DIRECTION('ref_axis',(0.,0.,-1.));
#26695=DIRECTION('center_axis',(1.,0.,0.));
#26696=DIRECTION('ref_axis',(0.,0.,-1.));
#26697=DIRECTION('',(0.,1.,0.));
#26698=DIRECTION('',(0.,0.,1.));
#26699=DIRECTION('center_axis',(1.,0.,0.));
#26700=DIRECTION('ref_axis',(0.,0.,-1.));
#26701=DIRECTION('center_axis',(0.,-1.,-1.22464679914735E-16));
#26702=DIRECTION('ref_axis',(0.,-1.22464679914735E-16,1.));
#26703=DIRECTION('center_axis',(1.,0.,0.));
#26704=DIRECTION('ref_axis',(0.,-1.,3.06161699786838E-17));
#26705=DIRECTION('center_axis',(1.,0.,0.));
#26706=DIRECTION('ref_axis',(0.,-1.,3.06161699786838E-17));
#26707=DIRECTION('center_axis',(1.,0.,0.));
#26708=DIRECTION('ref_axis',(0.,1.,0.));
#26709=DIRECTION('',(-0.707106781186545,0.70710678118655,8.65956056235496E-17));
#26710=DIRECTION('center_axis',(-1.,0.,0.));
#26711=DIRECTION('ref_axis',(0.,-1.,3.06161699786838E-17));
#26712=DIRECTION('center_axis',(-1.,0.,0.));
#26713=DIRECTION('ref_axis',(0.,-1.,3.06161699786838E-17));
#26714=DIRECTION('center_axis',(1.,0.,0.));
#26715=DIRECTION('ref_axis',(0.,0.,-1.));
#26716=DIRECTION('center_axis',(0.,-1.,-1.22464679914735E-16));
#26717=DIRECTION('ref_axis',(0.,-1.22464679914735E-16,1.));
#26718=DIRECTION('center_axis',(1.,0.,0.));
#26719=DIRECTION('ref_axis',(0.,-1.,1.83697019872103E-16));
#26720=DIRECTION('center_axis',(1.,0.,0.));
#26721=DIRECTION('ref_axis',(0.,-1.,1.83697019872103E-16));
#26722=DIRECTION('center_axis',(1.,0.,0.));
#26723=DIRECTION('ref_axis',(0.,1.,0.));
#26724=DIRECTION('',(-1.,0.,0.));
#26725=DIRECTION('center_axis',(1.,0.,0.));
#26726=DIRECTION('ref_axis',(0.,1.,-1.82855839818329E-16));
#26727=DIRECTION('center_axis',(1.,0.,0.));
#26728=DIRECTION('ref_axis',(0.,0.,-1.));
#26729=DIRECTION('center_axis',(0.,-3.05320519733064E-16,-1.));
#26730=DIRECTION('ref_axis',(0.,-1.,3.05320519733064E-16));
#26731=DIRECTION('center_axis',(1.,0.,0.));
#26732=DIRECTION('ref_axis',(0.,0.,-1.));
#26733=DIRECTION('center_axis',(0.,-1.,-1.22464679914735E-16));
#26734=DIRECTION('ref_axis',(0.,-1.22464679914735E-16,1.));
#26735=DIRECTION('center_axis',(1.,0.,0.));
#26736=DIRECTION('ref_axis',(0.,-1.,1.83697019872103E-16));
#26737=DIRECTION('center_axis',(-1.,0.,0.));
#26738=DIRECTION('ref_axis',(0.,0.,1.));
#26739=DIRECTION('center_axis',(-1.,0.,0.));
#26740=DIRECTION('ref_axis',(0.,-1.,1.83697019872103E-16));
#26741=DIRECTION('center_axis',(0.,0.,-1.));
#26742=DIRECTION('ref_axis',(-0.707106781186548,-0.707106781186548,0.));
#26743=DIRECTION('center_axis',(0.,0.,1.));
#26744=DIRECTION('ref_axis',(-1.,0.,0.));
#26745=DIRECTION('',(0.,0.,1.));
#26746=DIRECTION('center_axis',(-0.707106781186548,0.,-0.707106781186548));
#26747=DIRECTION('ref_axis',(-0.707106781186547,0.,0.707106781186547));
#26748=DIRECTION('center_axis',(0.408248290463865,-0.816496580927727,0.40824829046386));
#26749=DIRECTION('ref_axis',(-0.577350269189626,-0.577350269189627,-0.577350269189624));
#26750=DIRECTION('center_axis',(-1.,0.,0.));
#26751=DIRECTION('ref_axis',(0.,-0.707106781186546,-0.707106781186549));
#26752=DIRECTION('center_axis',(1.,0.,0.));
#26753=DIRECTION('ref_axis',(0.,-0.707106781186548,0.707106781186548));
#26754=DIRECTION('',(1.,0.,0.));
#26755=DIRECTION('center_axis',(1.,0.,0.));
#26756=DIRECTION('ref_axis',(0.,-1.,0.));
#26757=DIRECTION('',(-1.,0.,0.));
#26758=DIRECTION('center_axis',(0.,-1.,0.));
#26759=DIRECTION('ref_axis',(0.,0.,-1.));
#26760=DIRECTION('',(-1.,0.,0.));
#26761=DIRECTION('',(0.,0.,-1.));
#26762=DIRECTION('center_axis',(1.,0.,0.));
#26763=DIRECTION('ref_axis',(0.,-0.707106781186548,-0.707106781186548));
#26764=DIRECTION('center_axis',(1.,0.,0.));
#26765=DIRECTION('ref_axis',(0.,-0.707106781186546,-0.707106781186549));
#26766=DIRECTION('center_axis',(0.,1.,-1.63268091856641E-16));
#26767=DIRECTION('ref_axis',(0.,1.63268091856641E-16,1.));
#26768=DIRECTION('',(-1.,0.,0.));
#26769=DIRECTION('center_axis',(-0.408248290463865,-0.816496580927727,0.40824829046386));
#26770=DIRECTION('ref_axis',(0.577350269189626,-0.577350269189627,-0.577350269189624));
#26771=DIRECTION('center_axis',(0.,0.,-1.));
#26772=DIRECTION('ref_axis',(0.707106781186548,-0.707106781186548,0.));
#26773=DIRECTION('center_axis',(1.,0.,0.));
#26774=DIRECTION('ref_axis',(0.,0.707106781186548,0.707106781186548));
#26775=DIRECTION('',(1.,0.,0.));
#26776=DIRECTION('center_axis',(-0.408248290463864,-0.816496580927727,-0.40824829046386));
#26777=DIRECTION('ref_axis',(0.577350269189627,-0.577350269189628,0.577350269189623));
#26778=DIRECTION('center_axis',(0.,-1.,0.));
#26779=DIRECTION('ref_axis',(0.,0.,1.));
#26780=DIRECTION('center_axis',(0.,0.,1.));
#26781=DIRECTION('ref_axis',(1.,0.,0.));
#26782=DIRECTION('center_axis',(0.,0.,-1.));
#26783=DIRECTION('ref_axis',(0.707106781186548,-0.707106781186548,0.));
#26784=DIRECTION('center_axis',(0.,-1.,0.));
#26785=DIRECTION('ref_axis',(0.707106781186548,0.,0.707106781186548));
#26786=DIRECTION('',(0.,-1.,0.));
#26787=DIRECTION('center_axis',(1.,0.,0.));
#26788=DIRECTION('ref_axis',(0.,0.,-1.));
#26789=DIRECTION('center_axis',(0.,-1.,-1.22464679914735E-16));
#26790=DIRECTION('ref_axis',(0.,-1.22464679914735E-16,1.));
#26791=DIRECTION('center_axis',(1.,0.,0.));
#26792=DIRECTION('ref_axis',(0.,-1.,1.83697019872103E-16));
#26793=DIRECTION('center_axis',(1.,0.,0.));
#26794=DIRECTION('ref_axis',(0.,-1.,1.83697019872103E-16));
#26795=DIRECTION('center_axis',(1.,0.,0.));
#26796=DIRECTION('ref_axis',(0.,1.,0.));
#26797=DIRECTION('center_axis',(-1.,0.,0.));
#26798=DIRECTION('ref_axis',(0.,1.,0.));
#26799=DIRECTION('',(-1.,0.,0.));
#26800=DIRECTION('center_axis',(-1.,0.,0.));
#26801=DIRECTION('ref_axis',(0.,1.,0.));
#26802=DIRECTION('center_axis',(1.,0.,0.));
#26803=DIRECTION('ref_axis',(0.,0.,-1.));
#26804=DIRECTION('center_axis',(0.,-1.,-1.22464679914735E-16));
#26805=DIRECTION('ref_axis',(0.,-1.22464679914735E-16,1.));
#26806=DIRECTION('center_axis',(1.,0.,0.));
#26807=DIRECTION('ref_axis',(0.,1.,0.));
#26808=DIRECTION('center_axis',(-1.,0.,0.));
#26809=DIRECTION('ref_axis',(0.,0.,1.));
#26810=DIRECTION('center_axis',(1.,0.,0.));
#26811=DIRECTION('ref_axis',(0.,0.,-1.));
#26812=DIRECTION('center_axis',(1.,0.,0.));
#26813=DIRECTION('ref_axis',(0.,1.,0.));
#26814=DIRECTION('',(1.,0.,0.));
#26815=DIRECTION('center_axis',(0.,0.,1.));
#26816=DIRECTION('ref_axis',(0.,-1.,0.));
#26817=DIRECTION('center_axis',(0.,0.,-1.));
#26818=DIRECTION('ref_axis',(0.,1.,0.));
#26819=DIRECTION('center_axis',(0.,-1.,0.));
#26820=DIRECTION('ref_axis',(0.,0.,-1.));
#26821=DIRECTION('center_axis',(0.,0.,1.));
#26822=DIRECTION('ref_axis',(0.,-1.,0.));
#26823=DIRECTION('center_axis',(0.,1.,0.));
#26824=DIRECTION('ref_axis',(0.,0.,1.));
#26825=DIRECTION('center_axis',(0.,-1.63268091856641E-16,-1.));
#26826=DIRECTION('ref_axis',(0.,1.,-1.63268091856641E-16));
#62000=CARTESIAN_POINT('',(0.,0.,0.));
#62001=CARTESIAN_POINT('Origin',(-6.69999999999999,-19.75,2.6));
#62002=CARTESIAN_POINT('',(-7.09999999999999,-21.2403502950465,2.6));
#62003=CARTESIAN_POINT('',(-7.,-20.9392803321658,2.86457513110645));
#62004=CARTESIAN_POINT('Ctrl Pts',(-7.09999999999999,-21.2403502950465,
2.59999999999964));
#62005=CARTESIAN_POINT('Ctrl Pts',(-7.1,-21.2390201143488,2.61086673229779));
#62006=CARTESIAN_POINT('Ctrl Pts',(-7.09955586847657,-21.2371830675583,
2.62168006860561));
#62007=CARTESIAN_POINT('Ctrl Pts',(-7.09868849358987,-21.2348575067649,
2.63236487415456));
#62008=CARTESIAN_POINT('Ctrl Pts',(-7.09693748140351,-21.2301627832357,
2.65393481468648));
#62009=CARTESIAN_POINT('Ctrl Pts',(-7.09345958992832,-21.2235106692755,
2.67487809903275));
#62010=CARTESIAN_POINT('Ctrl Pts',(-7.08092182655856,-21.2013035537358,
2.72631763724185));
#62011=CARTESIAN_POINT('Ctrl Pts',(-7.06990173845251,-21.1830658893345,
2.75455791698437));
#62012=CARTESIAN_POINT('Ctrl Pts',(-7.04472545150511,-21.1345591360924,
2.80504815321184));
#62013=CARTESIAN_POINT('Ctrl Pts',(-7.03094322851031,-21.1040599206881,
2.8253852234994));
#62014=CARTESIAN_POINT('Ctrl Pts',(-7.0101394940111,-21.0367728935879,2.85316918621411));
#62015=CARTESIAN_POINT('Ctrl Pts',(-7.00306375646934,-21.0013304617958,
2.8610826404679));
#62016=CARTESIAN_POINT('Ctrl Pts',(-7.00027014871753,-20.9564045695961,
2.86426972203768));
#62017=CARTESIAN_POINT('Ctrl Pts',(-6.99999999947518,-20.9478389844979,
2.86457513170154));
#62018=CARTESIAN_POINT('Ctrl Pts',(-7.,-20.9392803321658,2.86457513110645));
#62019=CARTESIAN_POINT('',(-7.09999999999999,-21.9,2.6));
#62020=CARTESIAN_POINT('',(-7.09999999999999,-19.75,2.6));
#62021=CARTESIAN_POINT('',(-6.69999999999999,-21.9,3.));
#62022=CARTESIAN_POINT('Origin',(-6.69999999999999,-21.9,2.6));
#62023=CARTESIAN_POINT('',(-6.69999999999999,-19.3,3.));
#62024=CARTESIAN_POINT('',(-6.69999999999999,-19.75,3.));
#62025=CARTESIAN_POINT('',(-7.,-19.,2.86457513110648));
#62026=CARTESIAN_POINT('Origin',(-6.69999999999999,-19.3,2.6));
#62027=CARTESIAN_POINT('',(-7.,-19.75,2.86457513110645));
#62028=CARTESIAN_POINT('Origin',(-6.69999999999999,-21.9,1.5));
#62029=CARTESIAN_POINT('',(-6.69999999999999,-22.3,-2.6));
#62030=CARTESIAN_POINT('',(-6.69999999999999,-22.3,2.6));
#62031=CARTESIAN_POINT('',(-6.69999999999999,-22.3,1.5));
#62032=CARTESIAN_POINT('Origin',(-6.69999999999999,-21.9,2.6));
#62033=CARTESIAN_POINT('',(-7.09999999999999,-21.9,-3.));
#62034=CARTESIAN_POINT('',(-7.09999999999999,-21.9,1.5));
#62035=CARTESIAN_POINT('Origin',(-6.69999999999999,-21.9,-2.6));
#62036=CARTESIAN_POINT('Origin',(-3.89999999999999,-21.9,-2.6));
#62037=CARTESIAN_POINT('',(-3.89999999999999,-22.3,-2.6));
#62038=CARTESIAN_POINT('',(-3.49999999999999,-21.9,-2.6));
#62039=CARTESIAN_POINT('Origin',(-3.89999999999999,-21.9,-2.6));
#62040=CARTESIAN_POINT('',(-3.89999999999999,-21.9,-3.));
#62041=CARTESIAN_POINT('Origin',(-3.89999999999999,-21.9,-2.6));
#62042=CARTESIAN_POINT('Origin',(-3.89999999999999,-21.9,-2.6));
#62043=CARTESIAN_POINT('Origin',(-7.09999999999999,-21.9,-2.6));
#62044=CARTESIAN_POINT('',(-7.09999999999999,-21.9,-3.));
#62045=CARTESIAN_POINT('',(-7.09999999999999,-22.3,-2.6));
#62046=CARTESIAN_POINT('Origin',(-3.89999999999999,-21.45,-2.6));
#62047=CARTESIAN_POINT('',(-3.89999999999999,-19.3,-3.));
#62048=CARTESIAN_POINT('',(-3.49999999999999,-19.3,-2.6));
#62049=CARTESIAN_POINT('Origin',(-3.89999999999999,-19.3,-2.6));
#62050=CARTESIAN_POINT('',(-3.49999999999999,-21.45,-2.6));
#62051=CARTESIAN_POINT('',(-3.89999999999999,-21.45,-3.));
#62052=CARTESIAN_POINT('Origin',(-3.89999999999999,-19.3,-2.6));
#62053=CARTESIAN_POINT('',(-3.89999999999999,-18.9,-2.6));
#62054=CARTESIAN_POINT('Origin',(-3.89999999999999,-19.3,-2.6));
#62055=CARTESIAN_POINT('Origin',(-3.89999999999999,-19.3,-2.6));
#62056=CARTESIAN_POINT('Origin',(-3.89999999999999,-21.9,2.6));
#62057=CARTESIAN_POINT('',(-3.89999999999999,-22.3,2.6));
#62058=CARTESIAN_POINT('',(-3.49999999999999,-21.9,2.6));
#62059=CARTESIAN_POINT('Origin',(-3.89999999999999,-21.9,2.6));
#62060=CARTESIAN_POINT('',(-3.89999999999999,-21.9,3.));
#62061=CARTESIAN_POINT('Origin',(-3.89999999999999,-21.9,2.6));
#62062=CARTESIAN_POINT('Origin',(-3.89999999999999,-21.9,2.6));
#62063=CARTESIAN_POINT('Origin',(-3.89999999999999,-21.9,1.5));
#62064=CARTESIAN_POINT('',(-3.89999999999999,-22.3,1.5));
#62065=CARTESIAN_POINT('',(-3.49999999999999,-21.9,1.5));
#62066=CARTESIAN_POINT('Origin',(-6.69999999999999,-21.9,2.6));
#62067=CARTESIAN_POINT('Origin',(-6.69999999999999,-21.9,2.6));
#62068=CARTESIAN_POINT('Origin',(-7.09999999999999,-19.3,2.6));
#62069=CARTESIAN_POINT('',(-3.89999999999999,-19.3,3.));
#62070=CARTESIAN_POINT('',(-7.09999999999999,-19.3,3.));
#62071=CARTESIAN_POINT('',(-3.89999999999999,-18.9,2.6));
#62072=CARTESIAN_POINT('Origin',(-3.89999999999999,-19.3,2.6));
#62073=CARTESIAN_POINT('',(-7.,-18.9,2.6));
#62074=CARTESIAN_POINT('',(-7.09999999999999,-18.9,2.6));
#62075=CARTESIAN_POINT('Origin',(-7.,-19.3,2.6));
#62076=CARTESIAN_POINT('Origin',(-7.09999999999999,-18.9,3.));
#62077=CARTESIAN_POINT('',(-7.09999999999999,-21.9,3.));
#62078=CARTESIAN_POINT('',(-3.89999999999999,-19.75,3.));
#62079=CARTESIAN_POINT('Origin',(-7.09999999999999,-22.3,3.));
#62080=CARTESIAN_POINT('',(-7.09999999999999,-22.3,2.6));
#62081=CARTESIAN_POINT('Origin',(-7.09999999999999,-21.9,2.6));
#62082=CARTESIAN_POINT('Origin',(-7.09999999999999,-19.3,-2.6));
#62083=CARTESIAN_POINT('',(-7.,-19.3,-3.));
#62084=CARTESIAN_POINT('',(-7.09999999999999,-19.3,-3.));
#62085=CARTESIAN_POINT('',(-7.,-18.9,-2.6));
#62086=CARTESIAN_POINT('Origin',(-7.,-19.3,-2.6));
#62087=CARTESIAN_POINT('',(-7.09999999999999,-18.9,-2.6));
#62088=CARTESIAN_POINT('Origin',(-3.89999999999999,-19.3,2.6));
#62089=CARTESIAN_POINT('',(-3.49999999999999,-19.3,2.6));
#62090=CARTESIAN_POINT('Origin',(-3.89999999999999,-19.3,2.6));
#62091=CARTESIAN_POINT('Origin',(-3.89999999999999,-19.3,2.6));
#62092=CARTESIAN_POINT('Origin',(-3.89999999999999,-19.75,2.6));
#62093=CARTESIAN_POINT('',(-3.49999999999999,-19.75,2.6));
#62094=CARTESIAN_POINT('Origin',(-3.89999999999999,-19.3,-1.5));
#62095=CARTESIAN_POINT('',(-3.89999999999999,-18.9,-1.5));
#62096=CARTESIAN_POINT('',(-3.49999999999999,-19.3,-1.5));
#62097=CARTESIAN_POINT('Origin',(-3.49999999999999,-20.6,2.22044604925031E-15));
#62098=CARTESIAN_POINT('Origin',(-7.09999999999999,-20.6,2.22044604925031E-15));
#62099=CARTESIAN_POINT('',(-7.10000000571368,-21.1875548662612,-3.));
#62100=CARTESIAN_POINT('Origin',(-7.09999999999999,0.,0.));
#62101=CARTESIAN_POINT('',(-7.09999999999999,-21.45,-3.));
#62102=CARTESIAN_POINT('Origin',(-6.69999999999999,2.6,19.75));
#62103=CARTESIAN_POINT('',(-7.09999999999999,2.6,21.2403502950465));
#62104=CARTESIAN_POINT('',(-7.,2.86457513110645,20.9392803321658));
#62105=CARTESIAN_POINT('Ctrl Pts',(-7.09999999999999,2.59999999999964,21.2403502950465));
#62106=CARTESIAN_POINT('Ctrl Pts',(-7.1,2.61086673229779,21.2390201143488));
#62107=CARTESIAN_POINT('Ctrl Pts',(-7.09955586847657,2.62168006860561,21.2371830675583));
#62108=CARTESIAN_POINT('Ctrl Pts',(-7.09868849358987,2.63236487415455,21.2348575067649));
#62109=CARTESIAN_POINT('Ctrl Pts',(-7.09693748140351,2.65393481468647,21.2301627832357));
#62110=CARTESIAN_POINT('Ctrl Pts',(-7.09345958992833,2.67487809903273,21.2235106692755));
#62111=CARTESIAN_POINT('Ctrl Pts',(-7.08092182655855,2.72631763724185,21.2013035537358));
#62112=CARTESIAN_POINT('Ctrl Pts',(-7.06990173845251,2.75455791698437,21.1830658893345));
#62113=CARTESIAN_POINT('Ctrl Pts',(-7.0447254515051,2.80504815321185,21.1345591360924));
#62114=CARTESIAN_POINT('Ctrl Pts',(-7.0309432285103,2.8253852234994,21.1040599206881));
#62115=CARTESIAN_POINT('Ctrl Pts',(-7.0101394940111,2.85316918621411,21.0367728935879));
#62116=CARTESIAN_POINT('Ctrl Pts',(-7.00306375646934,2.8610826404679,21.0013304617958));
#62117=CARTESIAN_POINT('Ctrl Pts',(-7.00027014871753,2.86426972203768,20.9564045695961));
#62118=CARTESIAN_POINT('Ctrl Pts',(-6.99999999947518,2.86457513170154,20.9478389844979));
#62119=CARTESIAN_POINT('Ctrl Pts',(-7.,2.86457513110645,20.9392803321658));
#62120=CARTESIAN_POINT('',(-7.09999999999999,2.6,21.9));
#62121=CARTESIAN_POINT('',(-7.09999999999999,2.6,19.75));
#62122=CARTESIAN_POINT('',(-6.69999999999999,3.,21.9));
#62123=CARTESIAN_POINT('Origin',(-6.69999999999999,2.6,21.9));
#62124=CARTESIAN_POINT('',(-6.69999999999999,3.,19.3));
#62125=CARTESIAN_POINT('',(-6.69999999999999,3.,19.75));
#62126=CARTESIAN_POINT('',(-7.,2.86457513110643,19.));
#62127=CARTESIAN_POINT('Origin',(-6.69999999999999,2.6,19.3));
#62128=CARTESIAN_POINT('',(-7.,2.86457513110645,19.75));
#62129=CARTESIAN_POINT('Origin',(-3.89999999999999,1.5,21.9));
#62130=CARTESIAN_POINT('',(-3.89999999999999,-2.6,22.3));
#62131=CARTESIAN_POINT('',(-3.49999999999999,-2.6,21.9));
#62132=CARTESIAN_POINT('Origin',(-3.89999999999999,-2.6,21.9));
#62133=CARTESIAN_POINT('',(-3.49999999999999,2.6,21.9));
#62134=CARTESIAN_POINT('',(-3.49999999999999,1.5,21.9));
#62135=CARTESIAN_POINT('',(-3.89999999999999,2.6,22.3));
#62136=CARTESIAN_POINT('Origin',(-3.89999999999999,2.6,21.9));
#62137=CARTESIAN_POINT('',(-3.89999999999999,1.5,22.3));
#62138=CARTESIAN_POINT('Origin',(-3.89999999999999,2.6,21.9));
#62139=CARTESIAN_POINT('',(-3.89999999999999,3.,21.9));
#62140=CARTESIAN_POINT('Origin',(-3.89999999999999,2.6,21.9));
#62141=CARTESIAN_POINT('Origin',(-3.89999999999999,2.6,21.9));
#62142=CARTESIAN_POINT('Origin',(-6.69999999999999,1.5,21.9));
#62143=CARTESIAN_POINT('',(-6.69999999999999,-2.6,22.3));
#62144=CARTESIAN_POINT('',(-6.69999999999999,2.6,22.3));
#62145=CARTESIAN_POINT('',(-6.69999999999999,1.5,22.3));
#62146=CARTESIAN_POINT('Origin',(-6.69999999999999,2.6,21.9));
#62147=CARTESIAN_POINT('',(-7.09999999999999,-3.,21.9));
#62148=CARTESIAN_POINT('',(-7.09999999999999,1.5,21.9));
#62149=CARTESIAN_POINT('Origin',(-6.69999999999999,-2.6,21.9));
#62150=CARTESIAN_POINT('Origin',(-7.09999999999999,-2.6,21.9));
#62151=CARTESIAN_POINT('',(-3.89999999999999,-3.,21.9));
#62152=CARTESIAN_POINT('',(-7.09999999999999,-3.,21.9));
#62153=CARTESIAN_POINT('Origin',(-3.89999999999999,-2.6,21.9));
#62154=CARTESIAN_POINT('',(-7.09999999999999,-2.6,22.3));
#62155=CARTESIAN_POINT('Origin',(-3.89999999999999,-2.6,21.9));
#62156=CARTESIAN_POINT('Origin',(-3.89999999999999,-2.6,21.9));
#62157=CARTESIAN_POINT('Origin',(-6.69999999999999,2.6,21.9));
#62158=CARTESIAN_POINT('Origin',(-6.69999999999999,2.6,21.9));
#62159=CARTESIAN_POINT('Origin',(-7.09999999999999,2.6,19.3));
#62160=CARTESIAN_POINT('',(-3.89999999999999,3.,19.3));
#62161=CARTESIAN_POINT('',(-7.09999999999999,3.,19.3));
#62162=CARTESIAN_POINT('',(-3.89999999999999,2.6,18.9));
#62163=CARTESIAN_POINT('Origin',(-3.89999999999999,2.6,19.3));
#62164=CARTESIAN_POINT('',(-7.,2.6,18.9));
#62165=CARTESIAN_POINT('',(-7.09999999999999,2.6,18.9));
#62166=CARTESIAN_POINT('Origin',(-7.,2.6,19.3));
#62167=CARTESIAN_POINT('Origin',(-7.09999999999999,3.,18.9));
#62168=CARTESIAN_POINT('',(-7.09999999999999,3.,21.9));
#62169=CARTESIAN_POINT('',(-3.89999999999999,3.,19.75));
#62170=CARTESIAN_POINT('Origin',(-7.09999999999999,2.6,21.9));
#62171=CARTESIAN_POINT('',(-7.09999999999999,2.6,22.3));
#62172=CARTESIAN_POINT('Origin',(-3.89999999999999,-2.6,19.3));
#62173=CARTESIAN_POINT('',(-3.89999999999999,-3.,19.3));
#62174=CARTESIAN_POINT('',(-3.49999999999999,-2.6,19.3));
#62175=CARTESIAN_POINT('Origin',(-3.89999999999999,-2.6,19.3));
#62176=CARTESIAN_POINT('',(-3.89999999999999,-2.6,18.9));
#62177=CARTESIAN_POINT('Origin',(-3.89999999999999,-2.6,19.3));
#62178=CARTESIAN_POINT('Origin',(-3.89999999999999,-2.6,19.3));
#62179=CARTESIAN_POINT('Origin',(-7.09999999999999,-2.6,19.3));
#62180=CARTESIAN_POINT('',(-7.,-3.,19.3));
#62181=CARTESIAN_POINT('',(-7.,-2.6,18.9));
#62182=CARTESIAN_POINT('Origin',(-7.,-2.6,19.3));
#62183=CARTESIAN_POINT('',(-7.09999999999999,-2.6,18.9));
#62184=CARTESIAN_POINT('',(-7.09999999999999,-3.,19.3));
#62185=CARTESIAN_POINT('Origin',(-3.89999999999999,2.6,19.3));
#62186=CARTESIAN_POINT('',(-3.49999999999999,2.6,19.3));
#62187=CARTESIAN_POINT('Origin',(-3.89999999999999,2.6,19.3));
#62188=CARTESIAN_POINT('Origin',(-3.89999999999999,2.6,19.3));
#62189=CARTESIAN_POINT('Origin',(-3.89999999999999,2.6,19.75));
#62190=CARTESIAN_POINT('',(-3.49999999999999,2.6,19.75));
#62191=CARTESIAN_POINT('Origin',(-3.89999999999999,-1.5,19.3));
#62192=CARTESIAN_POINT('',(-3.49999999999999,-1.5,19.3));
#62193=CARTESIAN_POINT('',(-3.89999999999999,-1.5,18.9));
#62194=CARTESIAN_POINT('Origin',(-3.89999999999999,-2.6,21.45));
#62195=CARTESIAN_POINT('',(-3.89999999999999,-3.,21.45));
#62196=CARTESIAN_POINT('',(-3.49999999999999,-2.6,21.45));
#62197=CARTESIAN_POINT('Origin',(-3.49999999999999,1.11022302462516E-15,
20.6));
#62198=CARTESIAN_POINT('Origin',(-7.09999999999999,1.11022302462516E-15,
20.6));
#62199=CARTESIAN_POINT('',(-7.09999999999999,-2.62060817839527E-15,21.3988897061572));
#62200=CARTESIAN_POINT('Origin',(-7.09999999999999,0.,0.));
#62201=CARTESIAN_POINT('',(-7.10000000571368,-3.,21.1875548662612));
#62202=CARTESIAN_POINT('Origin',(-7.09999999999999,0.,0.));
#62203=CARTESIAN_POINT('',(-7.09999999999999,-3.,21.45));
#62204=CARTESIAN_POINT('Origin',(-3.89999999999999,21.9,-1.5));
#62205=CARTESIAN_POINT('',(-3.49999999999999,21.9,-2.6));
#62206=CARTESIAN_POINT('',(-3.89999999999999,22.3,-2.6));
#62207=CARTESIAN_POINT('Origin',(-3.89999999999999,21.9,-2.6));
#62208=CARTESIAN_POINT('',(-3.89999999999999,22.3,2.6));
#62209=CARTESIAN_POINT('',(-3.89999999999999,22.3,-1.5));
#62210=CARTESIAN_POINT('',(-3.49999999999999,21.9,2.6));
#62211=CARTESIAN_POINT('Origin',(-3.89999999999999,21.9,2.6));
#62212=CARTESIAN_POINT('',(-3.49999999999999,21.9,-1.5));
#62213=CARTESIAN_POINT('Origin',(-3.89999999999999,21.9,2.6));
#62214=CARTESIAN_POINT('',(-3.89999999999999,21.9,3.));
#62215=CARTESIAN_POINT('Origin',(-3.89999999999999,21.9,2.6));
#62216=CARTESIAN_POINT('Origin',(-3.89999999999999,21.9,2.6));
#62217=CARTESIAN_POINT('Origin',(-3.89999999999999,21.9,-2.6));
#62218=CARTESIAN_POINT('',(-3.89999999999999,21.9,-3.));
#62219=CARTESIAN_POINT('Origin',(-3.89999999999999,21.9,-2.6));
#62220=CARTESIAN_POINT('Origin',(-3.89999999999999,21.9,-2.6));
#62221=CARTESIAN_POINT('Origin',(-7.09999999999999,21.9,-2.6));
#62222=CARTESIAN_POINT('',(-6.69999999999999,21.9,-3.));
#62223=CARTESIAN_POINT('',(-7.09999999999999,21.9,-3.));
#62224=CARTESIAN_POINT('',(-6.69999999999999,22.3,-2.6));
#62225=CARTESIAN_POINT('Origin',(-6.69999999999999,21.9,-2.6));
#62226=CARTESIAN_POINT('',(-7.09999999999999,22.3,-2.6));
#62227=CARTESIAN_POINT('Origin',(-3.89999999999999,19.75,-2.6));
#62228=CARTESIAN_POINT('',(-3.49999999999999,19.3,-2.6));
#62229=CARTESIAN_POINT('',(-3.49999999999999,19.75,-2.6));
#62230=CARTESIAN_POINT('',(-3.89999999999999,19.3,-3.));
#62231=CARTESIAN_POINT('Origin',(-3.89999999999999,19.3,-2.6));
#62232=CARTESIAN_POINT('',(-3.89999999999999,19.75,-3.));
#62233=CARTESIAN_POINT('Origin',(-3.49999999999999,20.6,0.));
#62234=CARTESIAN_POINT('',(-3.49999999999999,19.3,2.6));
#62235=CARTESIAN_POINT('',(-3.49999999999999,21.45,2.6));
#62236=CARTESIAN_POINT('',(-3.49999999999999,19.3,1.5));
#62237=CARTESIAN_POINT('Origin',(-6.69999999999999,19.75,-2.6));
#62238=CARTESIAN_POINT('',(-7.09999999999999,21.2403502950465,-2.6));
#62239=CARTESIAN_POINT('',(-7.,20.9392803321658,-2.86457513110645));
#62240=CARTESIAN_POINT('Ctrl Pts',(-7.09999999999999,21.2403502950465,-2.59999999999964));
#62241=CARTESIAN_POINT('Ctrl Pts',(-7.1,21.2390201143488,-2.61086673229778));
#62242=CARTESIAN_POINT('Ctrl Pts',(-7.09955586847657,21.2371830675583,-2.6216800686056));
#62243=CARTESIAN_POINT('Ctrl Pts',(-7.09868849358987,21.2348575067649,-2.63236487415455));
#62244=CARTESIAN_POINT('Ctrl Pts',(-7.09693748140351,21.2301627832357,-2.6539348146865));
#62245=CARTESIAN_POINT('Ctrl Pts',(-7.09345958992831,21.2235106692755,-2.67487809903278));
#62246=CARTESIAN_POINT('Ctrl Pts',(-7.08092182655856,21.2013035537358,-2.72631763724183));
#62247=CARTESIAN_POINT('Ctrl Pts',(-7.06990173845252,21.1830658893345,-2.75455791698435));
#62248=CARTESIAN_POINT('Ctrl Pts',(-7.04472545150511,21.1345591360924,-2.80504815321183));
#62249=CARTESIAN_POINT('Ctrl Pts',(-7.03094322851031,21.1040599206881,-2.82538522349939));
#62250=CARTESIAN_POINT('Ctrl Pts',(-7.01013949401111,21.0367728935879,-2.8531691862141));
#62251=CARTESIAN_POINT('Ctrl Pts',(-7.00306375646934,21.0013304617958,-2.8610826404679));
#62252=CARTESIAN_POINT('Ctrl Pts',(-7.00027014871753,20.9564045695961,-2.86426972203768));
#62253=CARTESIAN_POINT('Ctrl Pts',(-6.99999999947518,20.9478389844979,-2.86457513170154));
#62254=CARTESIAN_POINT('Ctrl Pts',(-7.,20.9392803321658,-2.86457513110645));
#62255=CARTESIAN_POINT('',(-7.09999999999999,21.9,-2.6));
#62256=CARTESIAN_POINT('',(-7.09999999999999,19.75,-2.6));
#62257=CARTESIAN_POINT('Origin',(-6.69999999999999,21.9,-2.6));
#62258=CARTESIAN_POINT('',(-6.69999999999999,19.3,-3.));
#62259=CARTESIAN_POINT('',(-6.69999999999999,19.75,-3.));
#62260=CARTESIAN_POINT('',(-7.,19.,-2.86457513110643));
#62261=CARTESIAN_POINT('Origin',(-6.69999999999999,19.3,-2.6));
#62262=CARTESIAN_POINT('',(-7.,19.75,-2.86457513110645));
#62263=CARTESIAN_POINT('Origin',(-6.69999999999999,21.9,-1.5));
#62264=CARTESIAN_POINT('Origin',(-6.69999999999999,21.9,-2.6));
#62265=CARTESIAN_POINT('',(-7.09999999999999,21.9,2.6));
#62266=CARTESIAN_POINT('',(-7.09999999999999,21.9,-1.5));
#62267=CARTESIAN_POINT('',(-6.69999999999999,22.3,2.6));
#62268=CARTESIAN_POINT('Origin',(-6.69999999999999,21.9,2.6));
#62269=CARTESIAN_POINT('',(-6.69999999999999,22.3,-1.5));
#62270=CARTESIAN_POINT('Origin',(-6.69999999999999,21.45,2.6));
#62271=CARTESIAN_POINT('',(-7.,19.,2.86457513110643));
#62272=CARTESIAN_POINT('',(-6.69999999999999,19.3,3.));
#62273=CARTESIAN_POINT('Origin',(-6.69999999999999,19.3,2.6));
#62274=CARTESIAN_POINT('',(-6.69999999999999,21.9,3.));
#62275=CARTESIAN_POINT('',(-6.69999999999999,21.45,3.));
#62276=CARTESIAN_POINT('Origin',(-6.69999999999999,21.9,2.6));
#62277=CARTESIAN_POINT('',(-7.09999999999999,21.2403502950465,2.6));
#62278=CARTESIAN_POINT('',(-7.09999999999999,21.45,2.6));
#62279=CARTESIAN_POINT('',(-7.,20.939280330552,2.86457513110645));
#62280=CARTESIAN_POINT('Ctrl Pts',(-7.,20.9392803305521,2.86457513110645));
#62281=CARTESIAN_POINT('Ctrl Pts',(-6.9999999978217,20.9726487442632,2.86457513357641));
#62282=CARTESIAN_POINT('Ctrl Pts',(-7.00418879911678,21.0059157565623,2.86000991879761));
#62283=CARTESIAN_POINT('Ctrl Pts',(-7.01958904143543,21.0718993033474,2.84089197849509));
#62284=CARTESIAN_POINT('Ctrl Pts',(-7.03129369231811,21.1035538664428,2.82549715408756));
#62285=CARTESIAN_POINT('Ctrl Pts',(-7.05699818661693,21.160006242706,2.7822473587533));
#62286=CARTESIAN_POINT('Ctrl Pts',(-7.07049988125604,21.1834359928131,2.75458608787846));
#62287=CARTESIAN_POINT('Ctrl Pts',(-7.08973887000163,21.2168017558866,2.69454207075082));
#62288=CARTESIAN_POINT('Ctrl Pts',(-7.09610571805172,21.2279327022523,2.66418093757161));
#62289=CARTESIAN_POINT('Ctrl Pts',(-7.09868849358987,21.2348575067649,2.63236487415455));
#62290=CARTESIAN_POINT('Ctrl Pts',(-7.09954198702743,21.2371458493331,2.62185106800518));
#62291=CARTESIAN_POINT('Ctrl Pts',(-7.09998646943438,21.2389629679018,2.61120519714679));
#62292=CARTESIAN_POINT('Ctrl Pts',(-7.09999989834893,21.2403098710973,2.60032927350281));
#62293=CARTESIAN_POINT('Ctrl Pts',(-7.09999999999999,21.2403301414833,2.60016464182416));
#62294=CARTESIAN_POINT('Ctrl Pts',(-7.09999999999999,21.2403502950465,2.6));
#62295=CARTESIAN_POINT('',(-7.,21.45,2.86457513110645));
#62296=CARTESIAN_POINT('Origin',(-6.69999999999999,21.9,2.6));
#62297=CARTESIAN_POINT('Origin',(-6.69999999999999,21.9,2.6));
#62298=CARTESIAN_POINT('Origin',(-6.69999999999999,21.9,-2.6));
#62299=CARTESIAN_POINT('Origin',(-7.09999999999999,19.3,-2.6));
#62300=CARTESIAN_POINT('',(-7.09999999999999,19.3,-3.));
#62301=CARTESIAN_POINT('',(-3.89999999999999,18.9,-2.6));
#62302=CARTESIAN_POINT('Origin',(-3.89999999999999,19.3,-2.6));
#62303=CARTESIAN_POINT('',(-7.,18.9,-2.6));
#62304=CARTESIAN_POINT('',(-7.09999999999999,18.9,-2.6));
#62305=CARTESIAN_POINT('Origin',(-7.,19.3,-2.6));
#62306=CARTESIAN_POINT('Origin',(-7.09999999999999,18.9,-3.));
#62307=CARTESIAN_POINT('Origin',(-7.09999999999999,22.3,-3.));
#62308=CARTESIAN_POINT('',(-7.09999999999999,22.3,2.6));
#62309=CARTESIAN_POINT('Origin',(-7.09999999999999,21.9,2.6));
#62310=CARTESIAN_POINT('',(-7.09999999999999,21.9,3.));
#62311=CARTESIAN_POINT('Origin',(-7.09999999999999,22.3,3.));
#62312=CARTESIAN_POINT('',(-3.89999999999999,19.3,3.));
#62313=CARTESIAN_POINT('',(-7.09999999999999,19.3,3.));
#62314=CARTESIAN_POINT('',(-3.89999999999999,21.45,3.));
#62315=CARTESIAN_POINT('Origin',(-7.09999999999999,19.3,2.6));
#62316=CARTESIAN_POINT('',(-7.,18.9,2.6));
#62317=CARTESIAN_POINT('Origin',(-7.,19.3,2.6));
#62318=CARTESIAN_POINT('',(-3.89999999999999,18.9,2.6));
#62319=CARTESIAN_POINT('',(-7.09999999999999,18.9,2.6));
#62320=CARTESIAN_POINT('Origin',(-3.89999999999999,19.3,2.6));
#62321=CARTESIAN_POINT('Origin',(-7.4,0.,0.));
#62322=CARTESIAN_POINT('',(-7.,-3.,20.9203071812343));
#62323=CARTESIAN_POINT('Ctrl Pts',(-7.10000000898043,-3.,21.187554863459));
#62324=CARTESIAN_POINT('Ctrl Pts',(-7.0714456188059,-3.,21.1548542805031));
#62325=CARTESIAN_POINT('Ctrl Pts',(-7.04641393471848,-3.,21.113705953019));
#62326=CARTESIAN_POINT('Ctrl Pts',(-7.01162679116877,-3.,21.0292320043449));
#62327=CARTESIAN_POINT('Ctrl Pts',(-7.,-3.,20.9703351236358));
#62328=CARTESIAN_POINT('Ctrl Pts',(-7.,-3.,20.9203071812343));
#62329=CARTESIAN_POINT('',(-7.11715728752538,-2.62284531190034E-15,21.4171572875254));
#62330=CARTESIAN_POINT('Origin',(-7.4,-2.58820706965092E-15,21.1343145750508));
#62331=CARTESIAN_POINT('',(-7.11715728752538,-21.4171572875254,-2.62284531190034E-15));
#62332=CARTESIAN_POINT('Origin',(-7.11715728752538,-1.11022302462516E-15,
-1.11022302462516E-15));
#62333=CARTESIAN_POINT('Origin',(-7.11715728752538,-1.11022302462516E-15,
-1.11022302462516E-15));
#62334=CARTESIAN_POINT('Origin',(-7.,0.,0.));
#62335=CARTESIAN_POINT('Origin',(-7.09999999999999,0.,0.));
#62336=CARTESIAN_POINT('',(-7.,2.86457513110645,-20.9392803571529));
#62337=CARTESIAN_POINT('Origin',(-7.,0.,0.));
#62338=CARTESIAN_POINT('',(-7.09999999999999,2.6,-21.2403502950465));
#62339=CARTESIAN_POINT('Ctrl Pts',(-7.09999999999999,2.6,-21.2403502950465));
#62340=CARTESIAN_POINT('Ctrl Pts',(-7.09999999999999,2.6003921713453,-21.2403022899296));
#62341=CARTESIAN_POINT('Ctrl Pts',(-7.09999942325386,2.6007842840571,-21.2402536221204));
#62342=CARTESIAN_POINT('Ctrl Pts',(-7.09999630362454,2.60184507611363,-21.2401201486839));
#62343=CARTESIAN_POINT('Ctrl Pts',(-7.09999266043989,2.60251362028008,-21.240034081592));
#62344=CARTESIAN_POINT('Ctrl Pts',(-7.09997602470054,2.60460481765257,-21.2397587769154));
#62345=CARTESIAN_POINT('Ctrl Pts',(-7.09995712122886,2.60602658190596,-21.2395627811672));
#62346=CARTESIAN_POINT('Ctrl Pts',(-7.09977488248242,2.61581335410445,-21.2381530086686));
#62347=CARTESIAN_POINT('Ctrl Pts',(-7.09935699857395,2.62412985850796,-21.2366498678362));
#62348=CARTESIAN_POINT('Ctrl Pts',(-7.09868849358987,2.63236487415455,-21.2348575067649));
#62349=CARTESIAN_POINT('Ctrl Pts',(-7.09715565553086,2.6512472246232,-21.2307477404491));
#62350=CARTESIAN_POINT('Ctrl Pts',(-7.09430136895356,2.66965802332072,-21.225133614234));
#62351=CARTESIAN_POINT('Ctrl Pts',(-7.08497519397776,2.71137287081551,-21.2083557037175));
#62352=CARTESIAN_POINT('Ctrl Pts',(-7.0776055735118,2.73375616436245,-21.1960045404144));
#62353=CARTESIAN_POINT('Ctrl Pts',(-7.05934927081274,2.77755052489804,-21.1632306404314));
#62354=CARTESIAN_POINT('Ctrl Pts',(-7.04831649738891,2.7976105486174,-21.1421536207631));
#62355=CARTESIAN_POINT('Ctrl Pts',(-7.02658383602801,2.83193954938331,-21.0909146928277));
#62356=CARTESIAN_POINT('Ctrl Pts',(-7.01639288683744,2.84497738989315,-21.0607499422713));
#62357=CARTESIAN_POINT('Ctrl Pts',(-7.00341459029669,2.86082920681864,-20.9995815899696));
#62358=CARTESIAN_POINT('Ctrl Pts',(-6.99999999999998,2.86457513110647,-20.9694560416778));
#62359=CARTESIAN_POINT('Ctrl Pts',(-7.,2.86457513110645,-20.9392803571526));
#62360=CARTESIAN_POINT('',(-7.09999999999999,-2.6,-21.2403502950465));
#62361=CARTESIAN_POINT('Origin',(-7.09999999999999,0.,0.));
#62362=CARTESIAN_POINT('',(-7.,-2.86457513110646,-20.9392803571529));
#62363=CARTESIAN_POINT('Ctrl Pts',(-7.,-2.86457513110646,-20.9392803571526));
#62364=CARTESIAN_POINT('Ctrl Pts',(-6.99999999999998,-2.86457513110648,
-20.9618455210744));
#62365=CARTESIAN_POINT('Ctrl Pts',(-7.00189590232315,-2.86246650530523,
-20.9844202381741));
#62366=CARTESIAN_POINT('Ctrl Pts',(-7.01140185478759,-2.85122632172449,
-21.0436263038058));
#62367=CARTESIAN_POINT('Ctrl Pts',(-7.02201855971974,-2.83837640858004,
-21.0785265213582));
#62368=CARTESIAN_POINT('Ctrl Pts',(-7.04364595086458,-2.80538967801371,
-21.1319953593187));
#62369=CARTESIAN_POINT('Ctrl Pts',(-7.05354342289825,-2.78840016518533,
-21.1519891336581));
#62370=CARTESIAN_POINT('Ctrl Pts',(-7.0689762416833,-2.7551424923852,-21.1807205825222));
#62371=CARTESIAN_POINT('Ctrl Pts',(-7.07477587083774,-2.74074065264234,
-21.1908445906006));
#62372=CARTESIAN_POINT('Ctrl Pts',(-7.08922373671821,-2.69693339673472,
-21.2159198464697));
#62373=CARTESIAN_POINT('Ctrl Pts',(-7.09600316823805,-2.66544420312709,
-21.227657750983));
#62374=CARTESIAN_POINT('Ctrl Pts',(-7.09868849358987,-2.63236487415455,
-21.2348575067649));
#62375=CARTESIAN_POINT('Ctrl Pts',(-7.09936536158736,-2.62402683826439,
-21.2366722903163));
#62376=CARTESIAN_POINT('Ctrl Pts',(-7.09978524624839,-2.61560576952592,
-21.238190470791));
#62377=CARTESIAN_POINT('Ctrl Pts',(-7.09996050880447,-2.60578130232895,
-21.2395967409211));
#62378=CARTESIAN_POINT('Ctrl Pts',(-7.09997780022238,-2.60442682623069,
-21.2397826271377));
#62379=CARTESIAN_POINT('Ctrl Pts',(-7.09999323912115,-2.60241617783349,
-21.2400466815348));
#62380=CARTESIAN_POINT('Ctrl Pts',(-7.09999666166736,-2.60176080456852,
-21.2401308801099));
#62381=CARTESIAN_POINT('Ctrl Pts',(-7.09999949086643,-2.60073687963955,
-21.2402595033544));
#62382=CARTESIAN_POINT('Ctrl Pts',(-7.09999999999999,-2.60036846778023,
-21.2403051914481));
#62383=CARTESIAN_POINT('Ctrl Pts',(-7.09999999999999,-2.59999999999997,
-21.2403502950465));
#62384=CARTESIAN_POINT('',(-7.,-20.9203071812343,-3.));
#62385=CARTESIAN_POINT('Origin',(-7.,0.,0.));
#62386=CARTESIAN_POINT('Ctrl Pts',(-7.10000000898044,-21.187554863459,-3.));
#62387=CARTESIAN_POINT('Ctrl Pts',(-7.0714456188059,-21.1548542805032,-3.));
#62388=CARTESIAN_POINT('Ctrl Pts',(-7.04641393471848,-21.113705953019,-3.));
#62389=CARTESIAN_POINT('Ctrl Pts',(-7.01162679116877,-21.0292320043449,
-3.));
#62390=CARTESIAN_POINT('Ctrl Pts',(-7.,-20.9703351236358,-3.));
#62391=CARTESIAN_POINT('Ctrl Pts',(-7.,-20.9203071812343,-3.));
#62392=CARTESIAN_POINT('Origin',(-7.,0.,0.));
#62393=CARTESIAN_POINT('Origin',(-7.,7.05,0.));
#62394=CARTESIAN_POINT('',(-7.,-2.86457513110643,-19.));
#62395=CARTESIAN_POINT('',(-7.,-2.86457513110646,-19.75));
#62396=CARTESIAN_POINT('',(-7.,-2.6,-18.9));
#62397=CARTESIAN_POINT('Origin',(-7.,-2.6,-19.3));
#62398=CARTESIAN_POINT('',(-7.,2.6,-18.9));
#62399=CARTESIAN_POINT('',(-7.,5.025,-18.9));
#62400=CARTESIAN_POINT('',(-7.,2.86457513110645,-19.));
#62401=CARTESIAN_POINT('Origin',(-7.,2.6,-19.3));
#62402=CARTESIAN_POINT('',(-7.,2.86457513110645,-21.45));
#62403=CARTESIAN_POINT('',(-7.,18.9,1.5));
#62404=CARTESIAN_POINT('',(-7.,2.025,18.9));
#62405=CARTESIAN_POINT('',(-7.,-3.,11.15));
#62406=CARTESIAN_POINT('',(-7.,-18.9,-1.5));
#62407=CARTESIAN_POINT('',(-7.,-7.625,-3.));
#62408=CARTESIAN_POINT('',(-7.,-10.7968626966597,6.52035061571116E-16));
#62409=CARTESIAN_POINT('Origin',(-7.,0.,0.));
#62410=CARTESIAN_POINT('Origin',(-7.25,0.,0.));
#62411=CARTESIAN_POINT('',(-7.38284271247462,-21.6828427124746,-2.65538239242476E-15));
#62412=CARTESIAN_POINT('',(-7.25,-21.55,-2.63911385216255E-15));
#62413=CARTESIAN_POINT('',(-7.38284271247462,-2.65538239242476E-15,21.6828427124746));
#62414=CARTESIAN_POINT('Origin',(-7.38284271247462,0.,-3.31922799053094E-15));
#62415=CARTESIAN_POINT('Origin',(-7.38284271247462,0.,-3.31922799053094E-15));
#62416=CARTESIAN_POINT('Origin',(-10.4,0.,0.));
#62417=CARTESIAN_POINT('',(-10.,-2.76770176607302E-15,22.6));
#62418=CARTESIAN_POINT('Origin',(-10.,0.,0.));
#62419=CARTESIAN_POINT('',(-10.4,-2.81668763803891E-15,23.));
#62420=CARTESIAN_POINT('Origin',(-10.4,-2.76770176607302E-15,22.6));
#62421=CARTESIAN_POINT('',(-10.4,-23.,-2.81668763803891E-15));
#62422=CARTESIAN_POINT('Origin',(-10.4,0.,0.));
#62423=CARTESIAN_POINT('Origin',(-10.4,0.,0.));
#62424=CARTESIAN_POINT('Origin',(-11.45,0.,0.));
#62425=CARTESIAN_POINT('',(-12.7343145750508,-23.,-2.81668763803891E-15));
#62426=CARTESIAN_POINT('',(-11.45,-23.,-2.81668763803891E-15));
#62427=CARTESIAN_POINT('',(-12.7343145750508,-2.81668763803891E-15,23.));
#62428=CARTESIAN_POINT('Origin',(-12.7343145750508,0.,0.));
#62429=CARTESIAN_POINT('Origin',(-12.7343145750508,0.,0.));
#62430=CARTESIAN_POINT('Origin',(-10.,21.8,0.));
#62431=CARTESIAN_POINT('',(-10.,-21.8,-2.66973002214123E-15));
#62432=CARTESIAN_POINT('Origin',(-10.,0.,0.));
#62433=CARTESIAN_POINT('Origin',(-3.89999999999999,19.3,2.6));
#62434=CARTESIAN_POINT('Origin',(-3.89999999999999,19.3,2.6));
#62435=CARTESIAN_POINT('Origin',(-3.89999999999999,19.3,2.6));
#62436=CARTESIAN_POINT('Origin',(-3.89999999999999,19.3,1.5));
#62437=CARTESIAN_POINT('Origin',(-3.89999999999999,19.3,-2.6));
#62438=CARTESIAN_POINT('',(-3.89999999999999,18.9,1.5));
#62439=CARTESIAN_POINT('Origin',(-3.89999999999999,21.45,2.6));
#62440=CARTESIAN_POINT('Origin',(-3.89999999999999,19.3,-2.6));
#62441=CARTESIAN_POINT('Origin',(-7.09999999999999,20.6,0.));
#62442=CARTESIAN_POINT('Origin',(-7.09999999999999,18.9,3.));
#62443=CARTESIAN_POINT('Origin',(-6.69999999999999,2.6,-21.45));
#62444=CARTESIAN_POINT('',(-6.69999999999999,3.,-19.3));
#62445=CARTESIAN_POINT('Origin',(-6.69999999999999,2.6,-19.3));
#62446=CARTESIAN_POINT('',(-6.69999999999999,3.,-21.9));
#62447=CARTESIAN_POINT('',(-6.69999999999999,3.,-21.45));
#62448=CARTESIAN_POINT('',(-7.09999999999999,2.6,-21.9));
#62449=CARTESIAN_POINT('Origin',(-6.69999999999999,2.6,-21.9));
#62450=CARTESIAN_POINT('',(-7.09999999999999,2.6,-21.45));
#62451=CARTESIAN_POINT('Origin',(-7.09999999999999,2.6,-21.9));
#62452=CARTESIAN_POINT('',(-6.69999999999999,2.6,-22.3));
#62453=CARTESIAN_POINT('Origin',(-6.69999999999999,2.6,-21.9));
#62454=CARTESIAN_POINT('',(-3.89999999999999,3.,-21.9));
#62455=CARTESIAN_POINT('',(-7.09999999999999,3.,-21.9));
#62456=CARTESIAN_POINT('',(-3.89999999999999,2.6,-22.3));
#62457=CARTESIAN_POINT('Origin',(-3.89999999999999,2.6,-21.9));
#62458=CARTESIAN_POINT('',(-7.09999999999999,2.6,-22.3));
#62459=CARTESIAN_POINT('Origin',(-3.89999999999999,2.6,-21.45));
#62460=CARTESIAN_POINT('',(-3.49999999999999,2.6,-21.9));
#62461=CARTESIAN_POINT('Origin',(-3.89999999999999,2.6,-21.9));
#62462=CARTESIAN_POINT('',(-3.89999999999999,3.,-19.3));
#62463=CARTESIAN_POINT('',(-3.89999999999999,3.,-21.45));
#62464=CARTESIAN_POINT('',(-3.49999999999999,2.6,-19.3));
#62465=CARTESIAN_POINT('Origin',(-3.89999999999999,2.6,-19.3));
#62466=CARTESIAN_POINT('',(-3.49999999999999,2.6,-21.45));
#62467=CARTESIAN_POINT('Origin',(-3.89999999999999,2.6,-19.3));
#62468=CARTESIAN_POINT('',(-3.89999999999999,2.6,-18.9));
#62469=CARTESIAN_POINT('Origin',(-3.89999999999999,2.6,-19.3));
#62470=CARTESIAN_POINT('Origin',(-3.89999999999999,2.6,-19.3));
#62471=CARTESIAN_POINT('Origin',(-3.89999999999999,2.6,-21.9));
#62472=CARTESIAN_POINT('Origin',(-3.89999999999999,2.6,-21.9));
#62473=CARTESIAN_POINT('Origin',(-6.69999999999999,2.6,-21.9));
#62474=CARTESIAN_POINT('Origin',(-6.69999999999999,2.6,-21.9));
#62475=CARTESIAN_POINT('Origin',(-7.09999999999999,-3.88578058618805E-15,
-20.6));
#62476=CARTESIAN_POINT('',(-7.09999999999999,-2.6,-21.9));
#62477=CARTESIAN_POINT('',(-7.09999999999999,-1.5,-21.9));
#62478=CARTESIAN_POINT('',(-7.09999999999999,-2.6,-19.75));
#62479=CARTESIAN_POINT('Origin',(-6.69999999999999,-1.5,-21.9));
#62480=CARTESIAN_POINT('',(-6.69999999999999,-2.6,-22.3));
#62481=CARTESIAN_POINT('',(-6.69999999999999,-1.5,-22.3));
#62482=CARTESIAN_POINT('Origin',(-6.69999999999999,-2.6,-21.9));
#62483=CARTESIAN_POINT('Origin',(-7.09999999999999,-3.,-22.3));
#62484=CARTESIAN_POINT('',(-3.89999999999999,-2.6,-22.3));
#62485=CARTESIAN_POINT('',(-3.89999999999999,-1.5,-22.3));
#62486=CARTESIAN_POINT('',(-7.09999999999999,-2.6,-22.3));
#62487=CARTESIAN_POINT('Origin',(-3.89999999999999,-1.5,-21.9));
#62488=CARTESIAN_POINT('',(-3.49999999999999,-2.6,-21.9));
#62489=CARTESIAN_POINT('',(-3.49999999999999,-1.5,-21.9));
#62490=CARTESIAN_POINT('Origin',(-3.89999999999999,-2.6,-21.9));
#62491=CARTESIAN_POINT('Origin',(-3.49999999999999,-3.88578058618805E-15,
-20.6));
#62492=CARTESIAN_POINT('',(-3.49999999999999,-2.6,-19.3));
#62493=CARTESIAN_POINT('',(-3.49999999999999,1.5,-19.3));
#62494=CARTESIAN_POINT('',(-3.49999999999999,-2.6,-19.75));
#62495=CARTESIAN_POINT('Origin',(-12.7343145750508,0.,0.));
#62496=CARTESIAN_POINT('',(-13.0171572875254,-2.80234000832244E-15,22.8828427124746));
#62497=CARTESIAN_POINT('Origin',(-12.7343145750508,-2.76770176607302E-15,
22.6));
#62498=CARTESIAN_POINT('',(-13.0171572875254,-22.8828427124746,-2.80234000832244E-15));
#62499=CARTESIAN_POINT('Origin',(-13.0171572875254,0.,-3.50292501040305E-15));
#62500=CARTESIAN_POINT('Origin',(-13.0171572875254,0.,-3.50292501040305E-15));
#62501=CARTESIAN_POINT('Origin',(-13.2,0.,0.));
#62502=CARTESIAN_POINT('',(-13.3828427124746,-22.5171572875254,-2.75755645980654E-15));
#62503=CARTESIAN_POINT('',(-13.2,-22.7,-2.77994823406449E-15));
#62504=CARTESIAN_POINT('',(-13.3828427124746,-2.75755645980654E-15,22.5171572875254));
#62505=CARTESIAN_POINT('Origin',(-13.3828427124746,0.,-3.44694557475818E-15));
#62506=CARTESIAN_POINT('Origin',(-13.3828427124746,0.,-3.44694557475818E-15));
#62507=CARTESIAN_POINT('Origin',(-7.66568542494924,0.,0.));
#62508=CARTESIAN_POINT('',(-7.66568542494924,-2.66973002214123E-15,21.8));
#62509=CARTESIAN_POINT('Origin',(-7.66568542494924,-2.62074415017534E-15,
21.4));
#62510=CARTESIAN_POINT('',(-7.66568542494924,-21.8,-2.66973002214123E-15));
#62511=CARTESIAN_POINT('Origin',(-7.66568542494924,0.,0.));
#62512=CARTESIAN_POINT('Origin',(-7.66568542494924,0.,0.));
#62513=CARTESIAN_POINT('Origin',(-8.75,0.,0.));
#62514=CARTESIAN_POINT('',(-8.75,-21.8,-2.66973002214123E-15));
#62515=CARTESIAN_POINT('Origin',(-7.4,0.,0.));
#62516=CARTESIAN_POINT('',(-7.45,-10.4,3.17533340522386E-15));
#62517=CARTESIAN_POINT('Origin',(-7.45,0.,0.));
#62518=CARTESIAN_POINT('Origin',(-7.4,-10.7968626966597,3.29650373003067E-15));
#62519=CARTESIAN_POINT('Origin',(-13.1,0.,0.));
#62520=CARTESIAN_POINT('',(-13.5,-2.72291821755713E-15,22.2343145750508));
#62521=CARTESIAN_POINT('Origin',(-13.1,-2.72291821755713E-15,22.2343145750508));
#62522=CARTESIAN_POINT('Origin',(-13.5,0.,0.));
#62523=CARTESIAN_POINT('Origin',(-13.5,22.4,0.));
#62524=CARTESIAN_POINT('',(-13.5,-9.12361865364778E-16,7.45));
#62525=CARTESIAN_POINT('Origin',(-13.5,0.,0.));
#62526=CARTESIAN_POINT('Origin',(-6.69999999999999,-2.6,-19.75));
#62527=CARTESIAN_POINT('',(-6.69999999999999,-3.,-21.9));
#62528=CARTESIAN_POINT('Origin',(-6.69999999999999,-2.6,-21.9));
#62529=CARTESIAN_POINT('',(-6.69999999999999,-3.,-19.3));
#62530=CARTESIAN_POINT('',(-6.69999999999999,-3.,-19.75));
#62531=CARTESIAN_POINT('Origin',(-6.69999999999999,-2.6,-19.3));
#62532=CARTESIAN_POINT('Origin',(-6.69999999999999,-2.6,-21.9));
#62533=CARTESIAN_POINT('Origin',(-6.69999999999999,-2.6,-21.9));
#62534=CARTESIAN_POINT('Origin',(-7.09999999999999,-2.6,-19.3));
#62535=CARTESIAN_POINT('',(-3.89999999999999,-3.,-19.3));
#62536=CARTESIAN_POINT('',(-7.09999999999999,-3.,-19.3));
#62537=CARTESIAN_POINT('',(-3.89999999999999,-2.6,-18.9));
#62538=CARTESIAN_POINT('Origin',(-3.89999999999999,-2.6,-19.3));
#62539=CARTESIAN_POINT('',(-7.09999999999999,-2.6,-18.9));
#62540=CARTESIAN_POINT('Origin',(-7.09999999999999,-3.,-18.9));
#62541=CARTESIAN_POINT('',(-3.89999999999999,-3.,-21.9));
#62542=CARTESIAN_POINT('',(-7.09999999999999,-3.,-21.9));
#62543=CARTESIAN_POINT('',(-3.89999999999999,-3.,-19.75));
#62544=CARTESIAN_POINT('Origin',(-7.09999999999999,-2.6,-21.9));
#62545=CARTESIAN_POINT('Origin',(-3.89999999999999,-2.6,-21.9));
#62546=CARTESIAN_POINT('Origin',(-7.09999999999999,3.,-22.3));
#62547=CARTESIAN_POINT('',(-7.09999999999999,3.,-19.3));
#62548=CARTESIAN_POINT('Origin',(-3.89999999999999,-2.6,-21.9));
#62549=CARTESIAN_POINT('Origin',(-3.89999999999999,-2.6,-21.9));
#62550=CARTESIAN_POINT('Origin',(-7.09999999999999,2.6,-19.3));
#62551=CARTESIAN_POINT('',(-7.09999999999999,2.6,-18.9));
#62552=CARTESIAN_POINT('Origin',(-3.89999999999999,-2.6,-19.3));
#62553=CARTESIAN_POINT('Origin',(-3.89999999999999,-2.6,-19.3));
#62554=CARTESIAN_POINT('Origin',(-3.89999999999999,-2.6,-19.3));
#62555=CARTESIAN_POINT('Origin',(-3.89999999999999,-2.6,-19.75));
#62556=CARTESIAN_POINT('Origin',(-3.89999999999999,1.5,-19.3));
#62557=CARTESIAN_POINT('',(-3.89999999999999,1.5,-18.9));
#62558=CARTESIAN_POINT('Origin',(-13.1,0.,0.));
#62559=CARTESIAN_POINT('',(-13.1,-8.63375993398884E-16,7.05));
#62560=CARTESIAN_POINT('Origin',(-13.1,-9.12361865364778E-16,7.45));
#62561=CARTESIAN_POINT('',(-13.1,-7.05,-8.63375993398884E-16));
#62562=CARTESIAN_POINT('Origin',(-13.1,0.,0.));
#62563=CARTESIAN_POINT('Origin',(-13.1,0.,0.));
#62564=CARTESIAN_POINT('Origin',(-10.25,0.,0.));
#62565=CARTESIAN_POINT('',(-11.95,-7.05,8.63375993398884E-16));
#62566=CARTESIAN_POINT('',(-11.95,-8.63375993398884E-16,7.05));
#62567=CARTESIAN_POINT('Origin',(-11.95,0.,0.));
#62568=CARTESIAN_POINT('',(-10.25,-7.05,-8.63375993398884E-16));
#62569=CARTESIAN_POINT('Origin',(-11.95,0.,0.));
#62570=CARTESIAN_POINT('Origin',(-11.95,0.,0.));
#62571=CARTESIAN_POINT('',(-11.55,-9.12361865364778E-16,7.45));
#62572=CARTESIAN_POINT('Origin',(-11.95,-9.12361865364778E-16,7.45));
#62573=CARTESIAN_POINT('Origin',(-11.55,0.,0.));
#62574=CARTESIAN_POINT('Origin',(-11.55,10.4,0.));
#62575=CARTESIAN_POINT('',(-11.55,-10.4,-1.27363267111325E-15));
#62576=CARTESIAN_POINT('Origin',(-11.55,0.,0.));
#62577=CARTESIAN_POINT('Origin',(-9.5,0.,0.));
#62578=CARTESIAN_POINT('',(-9.5,-10.4,-1.27363267111325E-15));
#62579=CARTESIAN_POINT('Origin',(-7.09999999999999,3.,-18.9));
#62580=CARTESIAN_POINT('Origin',(-7.09999999999999,-3.,18.9));
#62581=CARTESIAN_POINT('Origin',(-7.09999999999999,-3.,22.3));
#62582=CARTESIAN_POINT('Origin',(-7.09999999999999,3.,22.3));
#62583=CARTESIAN_POINT('Origin',(-7.09999999999999,-18.9,-3.));
#62584=CARTESIAN_POINT('Origin',(-7.09999999999999,-22.3,-3.));
#65546=UNCERTAINTY_MEASURE_WITH_UNIT(LENGTH_MEASURE(0.01),#65564,
'DISTANCE_ACCURACY_VALUE',
'Maximum model space distance between geometric entities at asserted c
onnectivities');
#65550=UNCERTAINTY_MEASURE_WITH_UNIT(LENGTH_MEASURE(0.01),#65564,
'DISTANCE_ACCURACY_VALUE',
'Maximum model space distance between geometric entities at asserted c
onnectivities');
#65559=(
GEOMETRIC_REPRESENTATION_CONTEXT(3)
GLOBAL_UNCERTAINTY_ASSIGNED_CONTEXT((#65546))
GLOBAL_UNIT_ASSIGNED_CONTEXT((#65564,#65566,#65567))
REPRESENTATION_CONTEXT('','3D')
);
#65563=(
GEOMETRIC_REPRESENTATION_CONTEXT(3)
GLOBAL_UNCERTAINTY_ASSIGNED_CONTEXT((#65550))
GLOBAL_UNIT_ASSIGNED_CONTEXT((#65564,#65566,#65567))
REPRESENTATION_CONTEXT('','3D')
);
#65564=(
LENGTH_UNIT()
NAMED_UNIT(*)
SI_UNIT(.MILLI.,.METRE.)
);
#65566=(
NAMED_UNIT(*)
PLANE_ANGLE_UNIT()
SI_UNIT($,.RADIAN.)
);
#65567=(
NAMED_UNIT(*)
SI_UNIT($,.STERADIAN.)
SOLID_ANGLE_UNIT()
);
#65576=SHAPE_DEFINITION_REPRESENTATION(#65588,#65621);
#65588=PRODUCT_DEFINITION_SHAPE('',$,#65634);
#65621=SHAPE_REPRESENTATION('',(#21777),#65559);
#65625=PRODUCT_DEFINITION_CONTEXT('part definition',#65663,'design');
#65634=PRODUCT_DEFINITION('2026-10-10-05-45-28-951',
'08_Sliding_Clutch_Collar',#65646,#65625);
#65646=PRODUCT_DEFINITION_FORMATION('',$,#65673);
#65663=APPLICATION_CONTEXT(
'Core Data for Automotive Mechanical Design Process');
#65664=PRODUCT_CONTEXT('part definition',#65663,'mechanical');
#65673=PRODUCT('2026-10-10-05-45-28-951','08_Sliding_Clutch_Collar',$,(#65664));
#65796=COLOUR_RGB('Off White',0.89,0.88,0.83);
#65797=FILL_AREA_STYLE_COLOUR('',#65796);
#65798=FILL_AREA_STYLE('',(#65797));
#65799=SURFACE_STYLE_FILL_AREA(#65798);
#65800=SURFACE_SIDE_STYLE('',(#65799));
#65801=SURFACE_STYLE_USAGE(.BOTH.,#65800);
#65802=PRESENTATION_STYLE_ASSIGNMENT((#65801));
ENDSEC;
END-ISO-10303-21;
